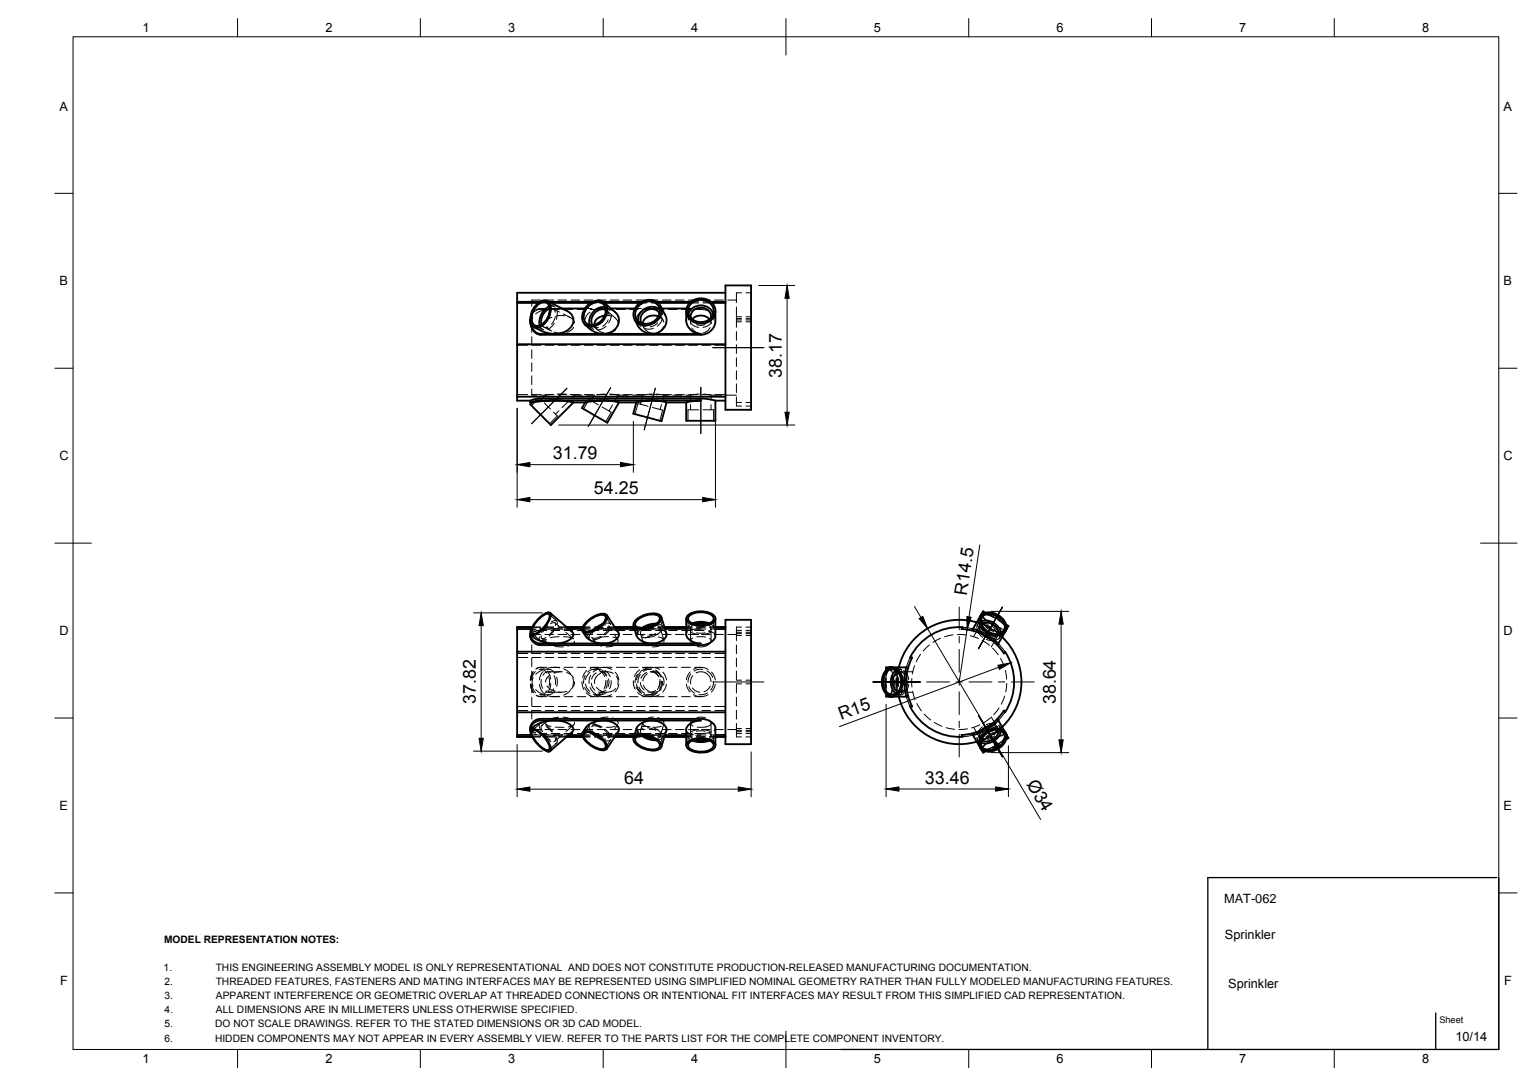
ISO-10303-21;
HEADER;
/* Generated by software containing ST-Developer
 * from STEP Tools, Inc. (www.steptools.com) 
 */

FILE_DESCRIPTION(
/* description */ (''),
/* implementation_level */ '2;1');

FILE_NAME(
/* name */ 'Sprinkler.step',
/* time_stamp */ '2026-10-24T10:18:25-07:00',
/* author */ (''),
/* organization */ (''),
/* preprocessor_version */ 'ST-DEVELOPER v20.2',
/* originating_system */ 'Autodesk Translation Framework v15.15.0.0',
/* authorisation */ '');

FILE_SCHEMA (('AUTOMOTIVE_DESIGN { 1 0 10303 214 3 1 1 }'));
ENDSEC;

DATA;
#10=MECHANICAL_DESIGN_GEOMETRIC_PRESENTATION_REPRESENTATION('',(#264),#14125);
#235=SHAPE_REPRESENTATION_RELATIONSHIP('SRR','None',#14209,#245);
#245=ADVANCED_BREP_SHAPE_REPRESENTATION('',(#277),#14123);
#264=STYLED_ITEM('',(#14263),#277);
#277=MANIFOLD_SOLID_BREP('Sprinkler',#6145);
#289=B_SPLINE_SURFACE_WITH_KNOTS('',3,1,((#13841,#13842),(#13843,#13844),
(#13845,#13846),(#13847,#13848),(#13849,#13850),(#13851,#13852),(#13853,
#13854),(#13855,#13856),(#13857,#13858),(#13859,#13860),(#13861,#13862)),
 .UNSPECIFIED.,.F.,.F.,.F.,(4,1,1,1,1,1,1,1,4),(2,2),(3.14159265358979,
3.53429173528852,3.92699081698724,4.31968989868597,4.71238898038469,5.10508806208341,
5.49778714378214,5.89048622548086,6.28318530717959),(0.,0.129347179873149),
 .UNSPECIFIED.);
#290=B_SPLINE_SURFACE_WITH_KNOTS('',3,1,((#13904,#13905),(#13906,#13907),
(#13908,#13909),(#13910,#13911),(#13912,#13913),(#13914,#13915),(#13916,
#13917),(#13918,#13919),(#13920,#13921),(#13922,#13923),(#13924,#13925)),
 .UNSPECIFIED.,.F.,.F.,.F.,(4,1,1,1,1,1,1,1,4),(2,2),(3.14159265358979,
3.53429173528851,3.92699081698724,4.31968989868596,4.71238898038469,5.10508806208341,
5.49778714378214,5.89048622548086,6.28318530717959),(0.,0.129347179873148),
 .UNSPECIFIED.);
#291=B_SPLINE_SURFACE_WITH_KNOTS('',3,1,((#13967,#13968),(#13969,#13970),
(#13971,#13972),(#13973,#13974),(#13975,#13976),(#13977,#13978),(#13979,
#13980),(#13981,#13982),(#13983,#13984),(#13985,#13986),(#13987,#13988)),
 .UNSPECIFIED.,.F.,.F.,.F.,(4,1,1,1,1,1,1,1,4),(2,2),(3.14159265358979,
3.53429173528851,3.92699081698723,4.31968989868596,4.71238898038468,5.10508806208341,
5.49778714378213,5.89048622548085,6.28318530717958),(0.,0.129347179873145),
 .UNSPECIFIED.);
#411=B_SPLINE_CURVE_WITH_KNOTS('',3,(#12350,#12351,#12352,#12353,#12354,
#12355,#12356,#12357),.UNSPECIFIED.,.F.,.F.,(4,2,2,4),(0.801601659973552,
0.908686694681274,1.06147652934293,1.21426636400458),.UNSPECIFIED.);
#412=B_SPLINE_CURVE_WITH_KNOTS('',3,(#12359,#12360,#12361,#12362,#12363,
#12364,#12365,#12366,#12367,#12368,#12369,#12370,#12371,#12372),
 .UNSPECIFIED.,.F.,.F.,(4,2,2,2,2,2,4),(0.,0.152789834661652,0.305579669323305,
0.456356425662796,0.607133182002287,0.757909938341781,0.801601659973552),
 .UNSPECIFIED.);
#413=B_SPLINE_CURVE_WITH_KNOTS('',3,(#12376,#12377,#12378,#12379,#12380,
#12381,#12382,#12383,#12384,#12385,#12386,#12387,#12388,#12389,#12390,#12391),
 .UNSPECIFIED.,.F.,.F.,(4,2,2,2,2,2,2,4),(1.41258149283994,1.51470567835646,
1.66615965590029,1.81761363344413,1.96906761098797,2.12052158853181,2.27200321656199,
2.42348484459217),.UNSPECIFIED.);
#414=B_SPLINE_CURVE_WITH_KNOTS('',3,(#12392,#12393,#12394,#12395,#12396,
#12397),.UNSPECIFIED.,.F.,.F.,(4,2,4),(1.21174242229609,1.36322405032627,
1.41258149283994),.UNSPECIFIED.);
#415=B_SPLINE_CURVE_WITH_KNOTS('',3,(#12402,#12403,#12404,#12405,#12406,
#12407,#12408,#12409),.UNSPECIFIED.,.F.,.F.,(4,2,2,4),(0.810459053731311,
0.931112082660273,1.09792489409666,1.26473770553305),.UNSPECIFIED.);
#416=B_SPLINE_CURVE_WITH_KNOTS('',3,(#12411,#12412,#12413,#12414,#12415,
#12416,#12417,#12418,#12419,#12420,#12421,#12422,#12423,#12424),
 .UNSPECIFIED.,.F.,.F.,(4,2,2,2,2,2,4),(0.,0.166812811436392,0.333625622872784,
0.482997237819655,0.632368852766526,0.781740467713401,0.810459053731311),
 .UNSPECIFIED.);
#417=B_SPLINE_CURVE_WITH_KNOTS('',3,(#12426,#12427,#12428,#12429,#12430,
#12431,#12432,#12433,#12434,#12435,#12436,#12437,#12438,#12439,#12440,#12441,
#12442,#12443),.UNSPECIFIED.,.F.,.F.,(4,2,2,2,2,2,2,2,4),(1.21426636400458,
1.37281902636882,1.53137168873306,1.68587949128402,1.84038729383497,1.99489509638593,
2.14940289893689,2.30795556130114,2.46650822366539),.UNSPECIFIED.);
#418=B_SPLINE_CURVE_WITH_KNOTS('',3,(#12448,#12449,#12450,#12451,#12452,
#12453,#12454,#12455,#12456,#12457),.UNSPECIFIED.,.F.,.F.,(4,2,2,2,4),(0.84921255840186,
0.855460999411689,1.0133776521287,1.20423317275903,1.39508869338936),
 .UNSPECIFIED.);
#419=B_SPLINE_CURVE_WITH_KNOTS('',3,(#12459,#12460,#12461,#12462,#12463,
#12464,#12465,#12466,#12467,#12468,#12469,#12470),.UNSPECIFIED.,.F.,.F.,
(4,2,2,2,2,4),(0.,0.19085552063033,0.38171104126066,0.539627693977667,0.697544346694674,
0.84921255840186),.UNSPECIFIED.);
#420=B_SPLINE_CURVE_WITH_KNOTS('',3,(#12472,#12473,#12474,#12475,#12476,
#12477,#12478,#12479,#12480,#12481,#12482,#12483,#12484,#12485,#12486,#12487,
#12488,#12489),.UNSPECIFIED.,.F.,.F.,(4,2,2,2,2,2,2,2,4),(1.26473770553305,
1.44115993597425,1.61758216641546,1.77878219205947,1.93998221770349,2.10118224334752,
2.26238226899155,2.43880449943275,2.61522672987395),.UNSPECIFIED.);
#421=B_SPLINE_CURVE_WITH_KNOTS('',3,(#12493,#12494,#12495,#12496,#12497,
#12498,#12499,#12500,#12501,#12502,#12503,#12504,#12505,#12506,#12507,#12508,
#12509,#12510,#12511,#12512,#12513,#12514),.UNSPECIFIED.,.F.,.F.,(4,2,2,
2,2,2,2,2,2,2,4),(1.39508869338936,1.63068735474474,1.86628601610013,2.01895939966093,
2.09529609144134,2.17163278322174,2.24796947500215,2.32430616678255,2.47697955034337,
2.71257821169876,2.94817687305416),.UNSPECIFIED.);
#422=B_SPLINE_CURVE_WITH_KNOTS('',3,(#12517,#12518,#12519,#12520,#12521,
#12522,#12523,#12524,#12525,#12526,#12527,#12528,#12529,#12530,#12531,#12532,
#12533,#12534,#12535,#12536,#12537,#12538,#12539,#12540,#12541,#12542),
 .UNSPECIFIED.,.F.,.F.,(4,2,2,2,2,2,2,2,2,2,2,2,4),(0.,0.0444658256706816,
0.109825747467382,0.210987273969983,0.363115011869221,0.476603266918211,
0.543343022865724,0.610052308554092,0.7232875236507,0.87579543247345,0.97697424211648,
1.04237097445545,1.08685368328188),.UNSPECIFIED.);
#423=B_SPLINE_CURVE_WITH_KNOTS('',3,(#12557,#12558,#12559,#12560,#12561,
#12562,#12563,#12564),.UNSPECIFIED.,.F.,.F.,(4,2,2,4),(0.801601659973551,
0.908686694681269,1.06147652934292,1.21426636400457),.UNSPECIFIED.);
#424=B_SPLINE_CURVE_WITH_KNOTS('',3,(#12566,#12567,#12568,#12569,#12570,
#12571,#12572,#12573,#12574,#12575,#12576,#12577,#12578,#12579),
 .UNSPECIFIED.,.F.,.F.,(4,2,2,2,2,2,4),(0.,0.152789834661651,0.305579669323302,
0.456356425662796,0.607133182002289,0.757909938341779,0.801601659973551),
 .UNSPECIFIED.);
#425=B_SPLINE_CURVE_WITH_KNOTS('',3,(#12583,#12584,#12585,#12586,#12587,
#12588,#12589,#12590,#12591,#12592,#12593,#12594,#12595,#12596,#12597,#12598),
 .UNSPECIFIED.,.F.,.F.,(4,2,2,2,2,2,2,4),(1.41258149283993,1.51470567835645,
1.66615965590029,1.81761363344413,1.96906761098797,2.1205215885318,2.27200321656199,
2.42348484459217),.UNSPECIFIED.);
#426=B_SPLINE_CURVE_WITH_KNOTS('',3,(#12599,#12600,#12601,#12602,#12603,
#12604),.UNSPECIFIED.,.F.,.F.,(4,2,4),(1.21174242229609,1.36322405032627,
1.41258149283993),.UNSPECIFIED.);
#427=B_SPLINE_CURVE_WITH_KNOTS('',3,(#12609,#12610,#12611,#12612,#12613,
#12614,#12615,#12616),.UNSPECIFIED.,.F.,.F.,(4,2,2,4),(0.810459053731318,
0.931112082660271,1.09792489409666,1.26473770553306),.UNSPECIFIED.);
#428=B_SPLINE_CURVE_WITH_KNOTS('',3,(#12618,#12619,#12620,#12621,#12622,
#12623,#12624,#12625,#12626,#12627,#12628,#12629,#12630,#12631),
 .UNSPECIFIED.,.F.,.F.,(4,2,2,2,2,2,4),(0.,0.166812811436393,0.333625622872785,
0.482997237819654,0.632368852766523,0.781740467713397,0.810459053731318),
 .UNSPECIFIED.);
#429=B_SPLINE_CURVE_WITH_KNOTS('',3,(#12633,#12634,#12635,#12636,#12637,
#12638,#12639,#12640,#12641,#12642,#12643,#12644,#12645,#12646,#12647,#12648,
#12649,#12650),.UNSPECIFIED.,.F.,.F.,(4,2,2,2,2,2,2,2,4),(1.21426636400457,
1.37281902636881,1.53137168873306,1.68587949128401,1.84038729383497,1.99489509638593,
2.14940289893689,2.30795556130114,2.46650822366538),.UNSPECIFIED.);
#430=B_SPLINE_CURVE_WITH_KNOTS('',3,(#12655,#12656,#12657,#12658,#12659,
#12660,#12661,#12662),.UNSPECIFIED.,.F.,.F.,(4,2,2,4),(0.848478832255458,
0.991796836691898,1.19347267089766,1.39514850510343),.UNSPECIFIED.);
#431=B_SPLINE_CURVE_WITH_KNOTS('',3,(#12664,#12665,#12666,#12667,#12668,
#12669,#12670,#12671,#12672,#12673,#12674,#12675,#12676,#12677),
 .UNSPECIFIED.,.F.,.F.,(4,2,2,2,2,2,4),(0.,0.201675834205757,0.403351668411514,
0.550462960481608,0.697574252551703,0.8446855446218,0.848478832255458),
 .UNSPECIFIED.);
#432=B_SPLINE_CURVE_WITH_KNOTS('',3,(#12679,#12680,#12681,#12682,#12683,
#12684,#12685,#12686,#12687,#12688,#12689,#12690,#12691,#12692,#12693,#12694,
#12695,#12696),.UNSPECIFIED.,.F.,.F.,(4,2,2,2,2,2,2,2,4),(1.26473770553306,
1.44115993597426,1.61758216641546,1.77878219205948,1.93998221770349,2.10118224334752,
2.26238226899154,2.43880449943275,2.61522672987395),.UNSPECIFIED.);
#433=B_SPLINE_CURVE_WITH_KNOTS('',3,(#12700,#12701,#12702,#12703,#12704,
#12705,#12706,#12707,#12708,#12709,#12710,#12711,#12712,#12713,#12714,#12715,
#12716,#12717,#12718,#12719,#12720,#12721),.UNSPECIFIED.,.F.,.F.,(4,2,2,
2,2,2,2,2,2,2,4),(1.39514850510343,1.60860320712188,1.82205790914033,1.99791237111712,
2.08583960210551,2.17376683309391,2.26169406408231,2.34962129507071,2.5254757570475,
2.73893045906596,2.95238516108442),.UNSPECIFIED.);
#434=B_SPLINE_CURVE_WITH_KNOTS('',3,(#12724,#12725,#12726,#12727,#12728,
#12729,#12730,#12731,#12732,#12733,#12734,#12735,#12736,#12737,#12738,#12739,
#12740,#12741,#12742,#12743,#12744,#12745,#12746,#12747,#12748,#12749),
 .UNSPECIFIED.,.F.,.F.,(4,2,2,2,2,2,2,2,2,2,2,2,4),(0.,0.0444658256707017,
0.109825747467453,0.210987273970143,0.363115011869592,0.4766032669186,0.543343022866364,
0.610052308555067,0.723287523653244,0.875795432478097,0.97697424212264,
1.04237097446268,1.08685368328966),.UNSPECIFIED.);
#435=B_SPLINE_CURVE_WITH_KNOTS('',3,(#12755,#12756,#12757,#12758,#12759,
#12760,#12761,#12762),.UNSPECIFIED.,.F.,.F.,(4,2,2,4),(0.80160165997355,
0.908686694681275,1.06147652934293,1.21426636400458),.UNSPECIFIED.);
#436=B_SPLINE_CURVE_WITH_KNOTS('',3,(#12764,#12765,#12766,#12767,#12768,
#12769,#12770,#12771,#12772,#12773,#12774,#12775,#12776,#12777),
 .UNSPECIFIED.,.F.,.F.,(4,2,2,2,2,2,4),(0.,0.152789834661653,0.305579669323305,
0.456356425662799,0.607133182002292,0.757909938341784,0.80160165997355),
 .UNSPECIFIED.);
#437=B_SPLINE_CURVE_WITH_KNOTS('',3,(#12781,#12782,#12783,#12784,#12785,
#12786,#12787,#12788,#12789,#12790,#12791,#12792,#12793,#12794,#12795,#12796),
 .UNSPECIFIED.,.F.,.F.,(4,2,2,2,2,2,2,4),(1.41258149283993,1.51470567835645,
1.66615965590029,1.81761363344413,1.96906761098797,2.12052158853181,2.27200321656199,
2.42348484459217),.UNSPECIFIED.);
#438=B_SPLINE_CURVE_WITH_KNOTS('',3,(#12797,#12798,#12799,#12800,#12801,
#12802),.UNSPECIFIED.,.F.,.F.,(4,2,4),(1.21174242229609,1.36322405032627,
1.41258149283993),.UNSPECIFIED.);
#439=B_SPLINE_CURVE_WITH_KNOTS('',3,(#12807,#12808,#12809,#12810,#12811,
#12812,#12813,#12814),.UNSPECIFIED.,.F.,.F.,(4,2,2,4),(0.810451797988797,
0.931104826917751,1.09791763835414,1.26473044979053),.UNSPECIFIED.);
#440=B_SPLINE_CURVE_WITH_KNOTS('',3,(#12816,#12817,#12818,#12819,#12820,
#12821,#12822,#12823,#12824,#12825,#12826,#12827,#12828,#12829),
 .UNSPECIFIED.,.F.,.F.,(4,2,2,2,2,2,4),(0.,0.163827053405726,0.327654106811452,
0.48000785191773,0.632361597024009,0.781733211970881,0.810451797988797),
 .UNSPECIFIED.);
#441=B_SPLINE_CURVE_WITH_KNOTS('',3,(#12831,#12832,#12833,#12834,#12835,
#12836,#12837,#12838,#12839,#12840,#12841,#12842,#12843,#12844,#12845,#12846,
#12847,#12848),.UNSPECIFIED.,.F.,.F.,(4,2,2,2,2,2,2,2,4),(1.21426636400458,
1.37281902636882,1.53137168873306,1.68587949128402,1.84038729383497,1.99489509638594,
2.1494028989369,2.30795556130114,2.46650822366539),.UNSPECIFIED.);
#442=B_SPLINE_CURVE_WITH_KNOTS('',3,(#12853,#12854,#12855,#12856,#12857,
#12858,#12859,#12860,#12861,#12862),.UNSPECIFIED.,.F.,.F.,(4,2,2,2,4),(0.849212558401863,
0.855460999411694,1.01337765212871,1.20423317275904,1.39508869338936),
 .UNSPECIFIED.);
#443=B_SPLINE_CURVE_WITH_KNOTS('',3,(#12864,#12865,#12866,#12867,#12868,
#12869,#12870,#12871,#12872,#12873,#12874,#12875),.UNSPECIFIED.,.F.,.F.,
(4,2,2,2,2,4),(0.,0.190855520630331,0.381711041260663,0.539627693977671,
0.697544346694678,0.849212558401863),.UNSPECIFIED.);
#444=B_SPLINE_CURVE_WITH_KNOTS('',3,(#12877,#12878,#12879,#12880,#12881,
#12882,#12883,#12884,#12885,#12886,#12887,#12888,#12889,#12890,#12891,#12892,
#12893,#12894),.UNSPECIFIED.,.F.,.F.,(4,2,2,2,2,2,2,2,4),(1.26473044979053,
1.45047293867533,1.63621542756013,1.78793284105988,1.93965025455964,2.0913676680594,
2.24308508155916,2.42882757044396,2.61457005932877),.UNSPECIFIED.);
#445=B_SPLINE_CURVE_WITH_KNOTS('',3,(#12898,#12899,#12900,#12901,#12902,
#12903,#12904,#12905,#12906,#12907,#12908,#12909,#12910,#12911,#12912,#12913,
#12914,#12915,#12916,#12917,#12918,#12919),.UNSPECIFIED.,.F.,.F.,(4,2,2,
2,2,2,2,2,2,2,4),(1.39508869338936,1.63068735474475,1.86628601610013,2.01895939966094,
2.09529609144135,2.17163278322175,2.24796947500216,2.32430616678257,2.47697955034339,
2.71257821169878,2.94817687305417),.UNSPECIFIED.);
#446=B_SPLINE_CURVE_WITH_KNOTS('',3,(#12922,#12923,#12924,#12925,#12926,
#12927,#12928,#12929,#12930,#12931,#12932,#12933,#12934,#12935,#12936,#12937,
#12938,#12939,#12940,#12941,#12942,#12943,#12944,#12945,#12946,#12947),
 .UNSPECIFIED.,.F.,.F.,(4,2,2,2,2,2,2,2,2,2,2,2,4),(0.,0.0444658256707104,
0.109825747467599,0.210987273970278,0.3631150118696,0.476603266918339,0.54334302286555,
0.610052308553677,0.723287523650531,0.875795432473984,0.97697424211741,
1.0423709744566,1.08685368328313),.UNSPECIFIED.);
#447=B_SPLINE_CURVE_WITH_KNOTS('',3,(#13048,#13049,#13050,#13051,#13052,
#13053,#13054,#13055,#13056,#13057,#13058,#13059,#13060,#13061,#13062,#13063,
#13064,#13065),.UNSPECIFIED.,.F.,.F.,(4,2,2,2,2,2,2,2,4),(-2.42440986895006,
-2.27286833474306,-2.12132680053607,-1.9698171011243,-1.81830740171254,
-1.66679770230078,-1.51528800288901,-1.36374646868202,-1.21220493447502),
 .UNSPECIFIED.);
#448=B_SPLINE_CURVE_WITH_KNOTS('',3,(#13115,#13116,#13117,#13118,#13119,
#13120,#13121,#13122,#13123,#13124,#13125,#13126,#13127,#13128,#13129,#13130,
#13131,#13132,#13133,#13134,#13135),.UNSPECIFIED.,.F.,.F.,(4,2,2,2,3,2,
2,2,2,4),(1.63431795680218,1.63484051213071,1.74655213492763,1.90358589296679,
2.06061965100595,2.19559646985844,2.33057328871092,2.44200600177385,2.55343871483678,
2.66004451397958),.UNSPECIFIED.);
#449=B_SPLINE_CURVE_WITH_KNOTS('',3,(#13136,#13137,#13138,#13139,#13140,
#13141,#13142,#13143,#13144,#13145,#13146,#13147,#13148,#13149,#13150,#13151,
#13152,#13153,#13154,#13155,#13156,#13157,#13158,#13159),.UNSPECIFIED.,
 .F.,.F.,(4,2,2,2,2,2,2,2,2,2,2,4),(2.66004451397958,2.66487142789972,2.77630414096266,
2.91128095981515,3.04625777866764,3.20329153670679,3.36032529474595,3.47203691754285,
3.5278927289413,3.58374854033975,3.63960435173821,3.69493760780813),
 .UNSPECIFIED.);
#450=B_SPLINE_CURVE_WITH_KNOTS('',3,(#13162,#13163,#13164,#13165,#13166,
#13167,#13168,#13169,#13170,#13171,#13172,#13173,#13174,#13175,#13176,#13177,
#13178,#13179,#13180,#13181,#13182,#13183,#13184),.UNSPECIFIED.,.F.,.F.,
(4,2,2,2,3,2,2,2,2,2,4),(1.63645246149242,1.6458071028209,1.76735674157733,
1.91500283165642,2.06264892173552,2.21065304350676,2.35865716527801,2.45711954510512,
2.55558192493224,2.65404430475936,2.66124396153498),.UNSPECIFIED.);
#451=B_SPLINE_CURVE_WITH_KNOTS('',3,(#13185,#13186,#13187,#13188,#13189,
#13190,#13191,#13192,#13193,#13194,#13195,#13196,#13197,#13198,#13199,#13200,
#13201,#13202,#13203,#13204,#13205,#13206),.UNSPECIFIED.,.F.,.F.,(4,2,2,
2,2,2,2,2,2,2,4),(2.66124396153498,2.75250668458648,2.90051080635773,3.04851492812899,
3.19616101820807,3.34380710828715,3.46535674704357,3.52613156642178,3.58690638579999,
3.64768120517821,3.69910138322794),.UNSPECIFIED.);
#452=B_SPLINE_CURVE_WITH_KNOTS('',3,(#13209,#13210,#13211,#13212,#13213,
#13214,#13215,#13216,#13217,#13218,#13219,#13220,#13221,#13222,#13223,#13224,
#13225,#13226,#13227,#13228,#13229),.UNSPECIFIED.,.F.,.F.,(4,2,2,3,2,2,
2,2,2,4),(1.48658026968319,1.57668032617585,1.70181043495793,1.82694054374001,
1.94229840394621,2.0576562641524,2.16466765320846,2.27167904226452,2.37869043132058,
2.39673280800115),.UNSPECIFIED.);
#453=B_SPLINE_CURVE_WITH_KNOTS('',3,(#13230,#13231,#13232,#13233,#13234,
#13235,#13236,#13237,#13238,#13239,#13240,#13241,#13242,#13243,#13244,#13245,
#13246,#13247,#13248,#13249),.UNSPECIFIED.,.F.,.F.,(4,2,2,2,2,2,2,2,2,4),
(2.39673280800115,2.48570182037664,2.60105968058284,2.71641754078903,2.84154764957111,
2.96667775835319,3.07591353624385,3.18514931413451,3.29438509202518,3.3135208134232),
 .UNSPECIFIED.);
#454=B_SPLINE_CURVE_WITH_KNOTS('',3,(#13252,#13253,#13254,#13255,#13256,
#13257,#13258,#13259,#13260,#13261,#13262,#13263,#13264,#13265,#13266,#13267,
#13268,#13269,#13270,#13271,#13272),.UNSPECIFIED.,.F.,.F.,(4,2,2,3,2,2,
2,2,2,4),(1.48667142164751,1.57677147814025,1.70190158692234,1.82703169570442,
1.94802136665288,2.06901103760135,2.17041340390623,2.27181577021112,2.37321813651602,
2.39644556681379),.UNSPECIFIED.);
#455=B_SPLINE_CURVE_WITH_KNOTS('',3,(#13273,#13274,#13275,#13276,#13277,
#13278,#13279,#13280,#13281,#13282,#13283,#13284,#13285,#13286,#13287,#13288,
#13289,#13290,#13291,#13292),.UNSPECIFIED.,.F.,.F.,(4,2,2,2,2,2,2,2,2,4),
(2.39644556681379,2.47462050282091,2.59561017376938,2.71659984471785,2.84172995349992,
2.966860062282,3.07609584017266,3.18533161806333,3.294567395954,3.31370311735193),
 .UNSPECIFIED.);
#456=B_SPLINE_CURVE_WITH_KNOTS('',3,(#13295,#13296,#13297,#13298,#13299,
#13300,#13301,#13302,#13303,#13304,#13305,#13306,#13307,#13308,#13309,#13310,
#13311,#13312,#13313,#13314,#13315),.UNSPECIFIED.,.F.,.F.,(4,2,2,3,2,2,
2,2,2,4),(1.42510602309759,1.50257240162674,1.61295870334865,1.72334500507057,
1.83225417045197,1.94116333583337,2.04500754168813,2.1488517475429,2.25269595339766,
2.2848744256183),.UNSPECIFIED.);
#457=B_SPLINE_CURVE_WITH_KNOTS('',3,(#13316,#13317,#13318,#13319,#13320,
#13321,#13322,#13323,#13324,#13325,#13326,#13327,#13328,#13329,#13330,#13331,
#13332,#13333,#13334,#13335),.UNSPECIFIED.,.F.,.F.,(4,2,2,2,2,2,2,2,2,4),
(2.2848744256183,2.35654015925242,2.46544932463382,2.57435849001523,2.68474479173714,
2.79513109345905,2.90282767176861,3.01052425007817,3.11822082838774,3.14845102816816),
 .UNSPECIFIED.);
#458=B_SPLINE_CURVE_WITH_KNOTS('',3,(#13338,#13339,#13340,#13341,#13342,
#13343,#13344,#13345,#13346,#13347,#13348,#13349,#13350,#13351,#13352,#13353,
#13354,#13355,#13356,#13357,#13358),.UNSPECIFIED.,.F.,.F.,(4,2,2,3,2,2,
2,2,2,4),(1.42506934481542,1.50220099251643,1.61276096598296,1.72332093944948,
1.83050112648501,1.93768131352053,2.04324956210919,2.14881781069785,2.25438605928651,
2.28497277338716),.UNSPECIFIED.);
#459=B_SPLINE_CURVE_WITH_KNOTS('',3,(#13359,#13360,#13361,#13362,#13363,
#13364,#13365,#13366,#13367,#13368,#13369,#13370,#13371,#13372,#13373,#13374,
#13375,#13376,#13377,#13378),.UNSPECIFIED.,.F.,.F.,(4,2,2,2,2,2,2,2,2,4),
(2.28497277338716,2.35995430787517,2.46713449491069,2.57431468194622,2.68487465541274,
2.79543462887926,2.90295645465092,3.01047828042258,3.11800010619425,3.1483902842649),
 .UNSPECIFIED.);
#460=B_SPLINE_CURVE_WITH_KNOTS('',3,(#13381,#13382,#13383,#13384,#13385,
#13386,#13387,#13388,#13389,#13390,#13391,#13392,#13393,#13394,#13395,#13396,
#13397,#13398,#13399,#13400),.UNSPECIFIED.,.F.,.F.,(4,2,2,2,2,2,2,2,2,4),
(0.140389663816896,0.211667950083815,0.317493899242379,0.423319848400943,
0.529145797559505,0.634971746718067,0.740805721759974,0.846639696801881,
0.952473671843789,0.987029360618753),.UNSPECIFIED.);
#461=B_SPLINE_CURVE_WITH_KNOTS('',3,(#13401,#13402,#13403,#13404,#13405,
#13406,#13407,#13408,#13409,#13410,#13411,#13412,#13413,#13414,#13415,#13416,
#13417,#13418,#13419,#13420,#13421),.UNSPECIFIED.,.F.,.F.,(4,2,2,2,2,2,
2,3,2,4),(0.987029360618753,1.0583076468857,1.16413359604426,1.26995954520282,
1.37578549436138,1.48161144351995,1.58744541856186,1.69327939360377,1.79911336864567,
1.83366905742066),.UNSPECIFIED.);
#462=B_SPLINE_CURVE_WITH_KNOTS('',3,(#13424,#13425,#13426,#13427,#13428,
#13429,#13430,#13431,#13432,#13433,#13434,#13435,#13436,#13437,#13438,#13439,
#13440,#13441,#13442,#13443),.UNSPECIFIED.,.F.,.F.,(4,2,2,2,2,2,2,2,2,4),
(0.14038966381692,0.211667950083817,0.317493899242381,0.423319848400946,
0.529145797559508,0.634971746718069,0.740805721759977,0.846639696801884,
0.952473671843792,0.987029360618756),.UNSPECIFIED.);
#463=B_SPLINE_CURVE_WITH_KNOTS('',3,(#13444,#13445,#13446,#13447,#13448,
#13449,#13450,#13451,#13452,#13453,#13454,#13455,#13456,#13457,#13458,#13459,
#13460,#13461,#13462,#13463,#13464),.UNSPECIFIED.,.F.,.F.,(4,2,2,2,2,2,
2,3,2,4),(0.987029360618756,1.0583076468857,1.16413359604426,1.26995954520282,
1.37578549436139,1.48161144351995,1.58744541856186,1.69327939360377,1.79911336864568,
1.83366905742069),.UNSPECIFIED.);
#464=B_SPLINE_CURVE_WITH_KNOTS('',3,(#13467,#13468,#13469,#13470,#13471,
#13472,#13473,#13474,#13475,#13476,#13477,#13478,#13479,#13480,#13481,#13482,
#13483,#13484,#13485,#13486,#13487),.UNSPECIFIED.,.F.,.F.,(4,2,2,2,3,2,
2,2,2,4),(1.63431795680214,1.63484051213073,1.74655213492764,1.90358589296679,
2.06061965100595,2.19559646985844,2.33057328871092,2.44200600177386,2.5534387148368,
2.66004451397959),.UNSPECIFIED.);
#465=B_SPLINE_CURVE_WITH_KNOTS('',3,(#13488,#13489,#13490,#13491,#13492,
#13493,#13494,#13495,#13496,#13497,#13498,#13499,#13500,#13501,#13502,#13503,
#13504,#13505,#13506,#13507,#13508,#13509,#13510,#13511),.UNSPECIFIED.,
 .F.,.F.,(4,2,2,2,2,2,2,2,2,2,2,4),(2.66004451397959,2.66487142789973,2.77630414096267,
2.91128095981515,3.04625777866764,3.2032915367068,3.36032529474595,3.47203691754286,
3.52789272894132,3.58374854033977,3.63960435173823,3.69493760780809),
 .UNSPECIFIED.);
#466=B_SPLINE_CURVE_WITH_KNOTS('',3,(#13514,#13515,#13516,#13517,#13518,
#13519,#13520,#13521,#13522,#13523,#13524,#13525,#13526,#13527,#13528,#13529,
#13530,#13531,#13532,#13533,#13534),.UNSPECIFIED.,.F.,.F.,(4,2,2,3,2,2,
2,2,2,4),(1.48658026968317,1.57668032617585,1.70181043495793,1.82694054374001,
1.9422984039462,2.0576562641524,2.16466765320846,2.27167904226452,2.37869043132058,
2.39673280800115),.UNSPECIFIED.);
#467=B_SPLINE_CURVE_WITH_KNOTS('',3,(#13535,#13536,#13537,#13538,#13539,
#13540,#13541,#13542,#13543,#13544,#13545,#13546,#13547,#13548,#13549,#13550,
#13551,#13552,#13553,#13554),.UNSPECIFIED.,.F.,.F.,(4,2,2,2,2,2,2,2,2,4),
(2.39673280800115,2.48570182037664,2.60105968058283,2.71641754078903,2.84154764957111,
2.96667775835319,3.07591353624386,3.18514931413453,3.29438509202519,3.31352081342317),
 .UNSPECIFIED.);
#468=B_SPLINE_CURVE_WITH_KNOTS('',3,(#13557,#13558,#13559,#13560,#13561,
#13562,#13563,#13564,#13565,#13566,#13567,#13568,#13569,#13570,#13571,#13572,
#13573,#13574,#13575,#13576,#13577),.UNSPECIFIED.,.F.,.F.,(4,2,2,3,2,2,
2,2,2,4),(1.42506934481545,1.50220099251643,1.61276096598296,1.72332093944948,
1.83050112648501,1.93768131352053,2.04324956210919,2.14881781069785,2.25438605928651,
2.28497277338716),.UNSPECIFIED.);
#469=B_SPLINE_CURVE_WITH_KNOTS('',3,(#13578,#13579,#13580,#13581,#13582,
#13583,#13584,#13585,#13586,#13587,#13588,#13589,#13590,#13591,#13592,#13593,
#13594,#13595,#13596,#13597),.UNSPECIFIED.,.F.,.F.,(4,2,2,2,2,2,2,2,2,4),
(2.28497277338716,2.35995430787516,2.46713449491069,2.57431468194622,2.68487465541274,
2.79543462887926,2.90295645465092,3.01047828042259,3.11800010619425,3.14839028426493),
 .UNSPECIFIED.);
#470=B_SPLINE_CURVE_WITH_KNOTS('',3,(#13600,#13601,#13602,#13603,#13604,
#13605,#13606,#13607,#13608,#13609,#13610,#13611,#13612,#13613,#13614,#13615,
#13616,#13617,#13618,#13619),.UNSPECIFIED.,.F.,.F.,(4,2,2,2,2,2,2,2,2,4),
(0.140389663816901,0.211667950083817,0.31749389924238,0.423319848400942,
0.529145797559504,0.634971746718067,0.740805721759975,0.846639696801883,
0.952473671843791,0.987029360618755),.UNSPECIFIED.);
#471=B_SPLINE_CURVE_WITH_KNOTS('',3,(#13620,#13621,#13622,#13623,#13624,
#13625,#13626,#13627,#13628,#13629,#13630,#13631,#13632,#13633,#13634,#13635,
#13636,#13637,#13638,#13639,#13640),.UNSPECIFIED.,.F.,.F.,(4,2,2,2,2,2,
2,3,2,4),(0.987029360618755,1.0583076468857,1.16413359604426,1.26995954520283,
1.37578549436139,1.48161144351995,1.58744541856186,1.69327939360377,1.79911336864568,
1.83366905742067),.UNSPECIFIED.);
#472=B_SPLINE_CURVE_WITH_KNOTS('',3,(#13667,#13668,#13669,#13670,#13671,
#13672,#13673,#13674,#13675,#13676,#13677,#13678,#13679,#13680,#13681,#13682,
#13683,#13684),.UNSPECIFIED.,.F.,.F.,(4,2,2,2,2,2,2,2,4),(-2.42440986895005,
-2.27286833474305,-2.12132680053606,-1.96981710112429,-1.81830740171253,
-1.66679770230077,-1.51528800288901,-1.36374646868202,-1.21220493447502),
 .UNSPECIFIED.);
#473=B_SPLINE_CURVE_WITH_KNOTS('',3,(#13696,#13697,#13698,#13699,#13700,
#13701,#13702,#13703,#13704,#13705,#13706,#13707,#13708,#13709,#13710,#13711,
#13712,#13713),.UNSPECIFIED.,.F.,.F.,(4,2,2,2,2,2,2,2,4),(-2.42440986895003,
-2.27286833474304,-2.12132680053605,-1.96981710112428,-1.81830740171252,
-1.66679770230076,-1.515288002889,-1.36374646868201,-1.21220493447502),
 .UNSPECIFIED.);
#474=B_SPLINE_CURVE_WITH_KNOTS('',3,(#13863,#13864,#13865,#13866,#13867,
#13868,#13869,#13870,#13871,#13872,#13873,#13874,#13875,#13876,#13877,#13878,
#13879,#13880,#13881,#13882,#13883,#13884,#13885,#13886,#13887,#13888,#13889,
#13890),.UNSPECIFIED.,.F.,.F.,(4,2,2,2,2,2,2,2,2,2,2,2,2,4),(-1.08391055751389,
-1.04041495858034,-0.976127049627852,-0.875975346180159,-0.713802892781725,
-0.606446034139209,-0.5422685089836,-0.478121096415875,-0.370996668444261,
-0.213675448646841,-0.11261366027741,-0.0448303332672381,-0.0212473968071398,
0.),.UNSPECIFIED.);
#475=B_SPLINE_CURVE_WITH_KNOTS('',3,(#13926,#13927,#13928,#13929,#13930,
#13931,#13932,#13933,#13934,#13935,#13936,#13937,#13938,#13939,#13940,#13941,
#13942,#13943,#13944,#13945,#13946,#13947,#13948,#13949,#13950,#13951,#13952,
#13953),.UNSPECIFIED.,.F.,.F.,(4,2,2,2,2,2,2,2,2,2,2,2,2,4),(-1.08391055750046,
-1.04041495856732,-0.976127049615459,-0.875975346168904,-0.713802892772233,
-0.606446034130957,-0.542268508976211,-0.478121096409307,-0.370996668439296,
-0.213675448644088,-0.112613660276149,-0.0448303332669679,-0.0212473968071859,
0.),.UNSPECIFIED.);
#476=B_SPLINE_CURVE_WITH_KNOTS('',3,(#13989,#13990,#13991,#13992,#13993,
#13994,#13995,#13996,#13997,#13998,#13999,#14000,#14001,#14002,#14003,#14004,
#14005,#14006,#14007,#14008,#14009,#14010,#14011,#14012,#14013,#14014,#14015,
#14016),.UNSPECIFIED.,.F.,.F.,(4,2,2,2,2,2,2,2,2,2,2,2,2,4),(-1.0839105575165,
-1.04041495858262,-0.976127049629671,-0.8759753461813,-0.713802892781876,
-0.606446034138857,-0.542268508983049,-0.478121096415206,-0.370996668443923,
-0.21367544864674,-0.112613660277534,-0.0448303332674202,-0.021247396807171,
0.),.UNSPECIFIED.);
#566=CYLINDRICAL_SURFACE('',#6670,15.);
#567=CYLINDRICAL_SURFACE('',#6673,15.);
#568=CYLINDRICAL_SURFACE('',#6676,15.);
#569=CYLINDRICAL_SURFACE('',#6679,15.);
#570=CYLINDRICAL_SURFACE('',#6680,15.);
#571=CYLINDRICAL_SURFACE('',#6681,15.);
#572=CYLINDRICAL_SURFACE('',#6682,15.);
#573=CYLINDRICAL_SURFACE('',#6683,15.);
#574=CYLINDRICAL_SURFACE('',#6686,15.);
#575=CYLINDRICAL_SURFACE('',#6687,15.);
#576=CYLINDRICAL_SURFACE('',#6688,15.);
#577=CYLINDRICAL_SURFACE('',#6689,15.);
#578=CYLINDRICAL_SURFACE('',#6690,15.);
#579=CYLINDRICAL_SURFACE('',#6691,15.);
#580=CYLINDRICAL_SURFACE('',#6692,15.);
#581=CYLINDRICAL_SURFACE('',#6693,15.);
#582=CYLINDRICAL_SURFACE('',#6694,15.);
#583=CYLINDRICAL_SURFACE('',#6697,15.);
#584=CYLINDRICAL_SURFACE('',#6707,17.);
#585=CYLINDRICAL_SURFACE('',#6717,4.00000000000012);
#586=CYLINDRICAL_SURFACE('',#6721,4.00000000000001);
#587=CYLINDRICAL_SURFACE('',#6725,4.00000000000001);
#588=CYLINDRICAL_SURFACE('',#6729,4.);
#589=CYLINDRICAL_SURFACE('',#6733,3.50000000000012);
#590=CYLINDRICAL_SURFACE('',#6737,3.5);
#591=CYLINDRICAL_SURFACE('',#6741,3.49999999999992);
#592=CYLINDRICAL_SURFACE('',#6742,12.9999999999984);
#593=CYLINDRICAL_SURFACE('',#6748,3.49999999999998);
#594=CYLINDRICAL_SURFACE('',#6749,2.80000000000012);
#595=CYLINDRICAL_SURFACE('',#6750,2.79999999999998);
#596=CYLINDRICAL_SURFACE('',#6751,2.79999999999991);
#597=CYLINDRICAL_SURFACE('',#6752,2.79999999999999);
#598=CYLINDRICAL_SURFACE('',#6756,4.00000000000012);
#599=CYLINDRICAL_SURFACE('',#6760,4.00000000000012);
#600=CYLINDRICAL_SURFACE('',#6764,4.00000000000001);
#601=CYLINDRICAL_SURFACE('',#6768,4.00000000000001);
#602=CYLINDRICAL_SURFACE('',#6772,4.00000000000001);
#603=CYLINDRICAL_SURFACE('',#6776,4.00000000000001);
#604=CYLINDRICAL_SURFACE('',#6780,4.);
#605=CYLINDRICAL_SURFACE('',#6784,4.);
#606=CYLINDRICAL_SURFACE('',#6785,2.80000000000012);
#607=CYLINDRICAL_SURFACE('',#6787,2.80000000000012);
#608=CYLINDRICAL_SURFACE('',#6789,2.79999999999998);
#609=CYLINDRICAL_SURFACE('',#6791,2.79999999999998);
#610=CYLINDRICAL_SURFACE('',#6793,2.79999999999991);
#611=CYLINDRICAL_SURFACE('',#6795,2.79999999999991);
#612=CYLINDRICAL_SURFACE('',#6797,2.79999999999999);
#613=CYLINDRICAL_SURFACE('',#6799,2.79999999999999);
#614=CYLINDRICAL_SURFACE('',#6803,3.50000000000012);
#615=CYLINDRICAL_SURFACE('',#6806,3.50000000000012);
#616=CYLINDRICAL_SURFACE('',#6809,3.5);
#617=CYLINDRICAL_SURFACE('',#6812,3.5);
#618=CYLINDRICAL_SURFACE('',#6815,3.49999999999992);
#619=CYLINDRICAL_SURFACE('',#6818,3.49999999999992);
#620=CYLINDRICAL_SURFACE('',#6821,3.49999999999998);
#621=CYLINDRICAL_SURFACE('',#6824,3.49999999999998);
#622=CYLINDRICAL_SURFACE('',#6829,14.5);
#623=CYLINDRICAL_SURFACE('',#6834,14.5);
#624=CYLINDRICAL_SURFACE('',#6839,14.5);
#687=FACE_BOUND('',#1399,.T.);
#688=FACE_BOUND('',#1401,.T.);
#689=FACE_BOUND('',#1404,.T.);
#690=FACE_BOUND('',#1407,.T.);
#691=FACE_BOUND('',#1410,.T.);
#692=FACE_BOUND('',#1413,.T.);
#693=FACE_BOUND('',#1416,.T.);
#694=FACE_BOUND('',#1419,.T.);
#695=FACE_BOUND('',#1422,.T.);
#696=FACE_BOUND('',#1425,.T.);
#697=FACE_BOUND('',#1428,.T.);
#698=FACE_BOUND('',#1429,.T.);
#699=FACE_BOUND('',#1430,.T.);
#700=FACE_BOUND('',#1431,.T.);
#701=FACE_BOUND('',#1432,.T.);
#702=FACE_BOUND('',#1433,.T.);
#703=FACE_BOUND('',#1434,.T.);
#704=FACE_BOUND('',#1435,.T.);
#705=FACE_BOUND('',#1436,.T.);
#706=FACE_BOUND('',#1437,.T.);
#707=FACE_BOUND('',#1438,.T.);
#708=FACE_BOUND('',#1439,.T.);
#709=FACE_BOUND('',#1442,.T.);
#710=FACE_BOUND('',#1449,.T.);
#711=FACE_BOUND('',#1452,.T.);
#712=FACE_BOUND('',#1455,.T.);
#713=FACE_BOUND('',#1458,.T.);
#714=FACE_BOUND('',#1461,.T.);
#715=FACE_BOUND('',#1464,.T.);
#716=FACE_BOUND('',#1467,.T.);
#717=FACE_BOUND('',#1470,.T.);
#718=FACE_BOUND('',#1481,.T.);
#719=FACE_BOUND('',#1484,.T.);
#720=FACE_BOUND('',#1487,.T.);
#721=FACE_BOUND('',#1490,.T.);
#722=FACE_BOUND('',#1493,.T.);
#723=FACE_BOUND('',#1496,.T.);
#724=FACE_BOUND('',#1499,.T.);
#725=FACE_BOUND('',#1502,.T.);
#726=FACE_BOUND('',#1510,.T.);
#727=FACE_BOUND('',#1517,.T.);
#728=FACE_BOUND('',#1524,.T.);
#967=FACE_OUTER_BOUND('',#1380,.T.);
#968=FACE_OUTER_BOUND('',#1381,.T.);
#969=FACE_OUTER_BOUND('',#1382,.T.);
#970=FACE_OUTER_BOUND('',#1383,.T.);
#971=FACE_OUTER_BOUND('',#1384,.T.);
#972=FACE_OUTER_BOUND('',#1385,.T.);
#973=FACE_OUTER_BOUND('',#1386,.T.);
#974=FACE_OUTER_BOUND('',#1387,.T.);
#975=FACE_OUTER_BOUND('',#1388,.T.);
#976=FACE_OUTER_BOUND('',#1389,.T.);
#977=FACE_OUTER_BOUND('',#1390,.T.);
#978=FACE_OUTER_BOUND('',#1391,.T.);
#979=FACE_OUTER_BOUND('',#1392,.T.);
#980=FACE_OUTER_BOUND('',#1393,.T.);
#981=FACE_OUTER_BOUND('',#1394,.T.);
#982=FACE_OUTER_BOUND('',#1395,.T.);
#983=FACE_OUTER_BOUND('',#1396,.T.);
#984=FACE_OUTER_BOUND('',#1397,.T.);
#985=FACE_OUTER_BOUND('',#1398,.T.);
#986=FACE_OUTER_BOUND('',#1400,.T.);
#987=FACE_OUTER_BOUND('',#1402,.T.);
#988=FACE_OUTER_BOUND('',#1403,.T.);
#989=FACE_OUTER_BOUND('',#1405,.T.);
#990=FACE_OUTER_BOUND('',#1406,.T.);
#991=FACE_OUTER_BOUND('',#1408,.T.);
#992=FACE_OUTER_BOUND('',#1409,.T.);
#993=FACE_OUTER_BOUND('',#1411,.T.);
#994=FACE_OUTER_BOUND('',#1412,.T.);
#995=FACE_OUTER_BOUND('',#1414,.T.);
#996=FACE_OUTER_BOUND('',#1415,.T.);
#997=FACE_OUTER_BOUND('',#1417,.T.);
#998=FACE_OUTER_BOUND('',#1418,.T.);
#999=FACE_OUTER_BOUND('',#1420,.T.);
#1000=FACE_OUTER_BOUND('',#1421,.T.);
#1001=FACE_OUTER_BOUND('',#1423,.T.);
#1002=FACE_OUTER_BOUND('',#1424,.T.);
#1003=FACE_OUTER_BOUND('',#1426,.T.);
#1004=FACE_OUTER_BOUND('',#1427,.T.);
#1005=FACE_OUTER_BOUND('',#1440,.T.);
#1006=FACE_OUTER_BOUND('',#1441,.T.);
#1007=FACE_OUTER_BOUND('',#1443,.T.);
#1008=FACE_OUTER_BOUND('',#1444,.T.);
#1009=FACE_OUTER_BOUND('',#1445,.T.);
#1010=FACE_OUTER_BOUND('',#1446,.T.);
#1011=FACE_OUTER_BOUND('',#1447,.T.);
#1012=FACE_OUTER_BOUND('',#1448,.T.);
#1013=FACE_OUTER_BOUND('',#1450,.T.);
#1014=FACE_OUTER_BOUND('',#1451,.T.);
#1015=FACE_OUTER_BOUND('',#1453,.T.);
#1016=FACE_OUTER_BOUND('',#1454,.T.);
#1017=FACE_OUTER_BOUND('',#1456,.T.);
#1018=FACE_OUTER_BOUND('',#1457,.T.);
#1019=FACE_OUTER_BOUND('',#1459,.T.);
#1020=FACE_OUTER_BOUND('',#1460,.T.);
#1021=FACE_OUTER_BOUND('',#1462,.T.);
#1022=FACE_OUTER_BOUND('',#1463,.T.);
#1023=FACE_OUTER_BOUND('',#1465,.T.);
#1024=FACE_OUTER_BOUND('',#1466,.T.);
#1025=FACE_OUTER_BOUND('',#1468,.T.);
#1026=FACE_OUTER_BOUND('',#1469,.T.);
#1027=FACE_OUTER_BOUND('',#1471,.T.);
#1028=FACE_OUTER_BOUND('',#1472,.T.);
#1029=FACE_OUTER_BOUND('',#1473,.T.);
#1030=FACE_OUTER_BOUND('',#1474,.T.);
#1031=FACE_OUTER_BOUND('',#1475,.T.);
#1032=FACE_OUTER_BOUND('',#1476,.T.);
#1033=FACE_OUTER_BOUND('',#1477,.T.);
#1034=FACE_OUTER_BOUND('',#1478,.T.);
#1035=FACE_OUTER_BOUND('',#1479,.T.);
#1036=FACE_OUTER_BOUND('',#1480,.T.);
#1037=FACE_OUTER_BOUND('',#1482,.T.);
#1038=FACE_OUTER_BOUND('',#1483,.T.);
#1039=FACE_OUTER_BOUND('',#1485,.T.);
#1040=FACE_OUTER_BOUND('',#1486,.T.);
#1041=FACE_OUTER_BOUND('',#1488,.T.);
#1042=FACE_OUTER_BOUND('',#1489,.T.);
#1043=FACE_OUTER_BOUND('',#1491,.T.);
#1044=FACE_OUTER_BOUND('',#1492,.T.);
#1045=FACE_OUTER_BOUND('',#1494,.T.);
#1046=FACE_OUTER_BOUND('',#1495,.T.);
#1047=FACE_OUTER_BOUND('',#1497,.T.);
#1048=FACE_OUTER_BOUND('',#1498,.T.);
#1049=FACE_OUTER_BOUND('',#1500,.T.);
#1050=FACE_OUTER_BOUND('',#1501,.T.);
#1051=FACE_OUTER_BOUND('',#1503,.T.);
#1052=FACE_OUTER_BOUND('',#1504,.T.);
#1053=FACE_OUTER_BOUND('',#1505,.T.);
#1054=FACE_OUTER_BOUND('',#1506,.T.);
#1055=FACE_OUTER_BOUND('',#1507,.T.);
#1056=FACE_OUTER_BOUND('',#1508,.T.);
#1057=FACE_OUTER_BOUND('',#1509,.T.);
#1058=FACE_OUTER_BOUND('',#1511,.T.);
#1059=FACE_OUTER_BOUND('',#1512,.T.);
#1060=FACE_OUTER_BOUND('',#1513,.T.);
#1061=FACE_OUTER_BOUND('',#1514,.T.);
#1062=FACE_OUTER_BOUND('',#1515,.T.);
#1063=FACE_OUTER_BOUND('',#1516,.T.);
#1064=FACE_OUTER_BOUND('',#1518,.T.);
#1065=FACE_OUTER_BOUND('',#1519,.T.);
#1066=FACE_OUTER_BOUND('',#1520,.T.);
#1067=FACE_OUTER_BOUND('',#1521,.T.);
#1068=FACE_OUTER_BOUND('',#1522,.T.);
#1069=FACE_OUTER_BOUND('',#1523,.T.);
#1070=FACE_OUTER_BOUND('',#1525,.T.);
#1071=FACE_OUTER_BOUND('',#1526,.T.);
#1072=FACE_OUTER_BOUND('',#1527,.T.);
#1073=FACE_OUTER_BOUND('',#1528,.T.);
#1074=FACE_OUTER_BOUND('',#1529,.T.);
#1075=FACE_OUTER_BOUND('',#1530,.T.);
#1076=FACE_OUTER_BOUND('',#1531,.T.);
#1077=FACE_OUTER_BOUND('',#1532,.T.);
#1078=FACE_OUTER_BOUND('',#1533,.T.);
#1380=EDGE_LOOP('',(#5069,#5070,#5071,#5072));
#1381=EDGE_LOOP('',(#5073,#5074,#5075,#5076));
#1382=EDGE_LOOP('',(#5077,#5078,#5079,#5080));
#1383=EDGE_LOOP('',(#5081,#5082,#5083,#5084,#5085,#5086));
#1384=EDGE_LOOP('',(#5087,#5088,#5089,#5090,#5091));
#1385=EDGE_LOOP('',(#5092,#5093,#5094,#5095,#5096));
#1386=EDGE_LOOP('',(#5097,#5098,#5099,#5100));
#1387=EDGE_LOOP('',(#5101,#5102,#5103,#5104));
#1388=EDGE_LOOP('',(#5105,#5106,#5107,#5108,#5109,#5110));
#1389=EDGE_LOOP('',(#5111,#5112,#5113,#5114,#5115));
#1390=EDGE_LOOP('',(#5116,#5117,#5118,#5119,#5120));
#1391=EDGE_LOOP('',(#5121,#5122,#5123,#5124));
#1392=EDGE_LOOP('',(#5125,#5126,#5127,#5128,#5129,#5130));
#1393=EDGE_LOOP('',(#5131,#5132,#5133,#5134,#5135));
#1394=EDGE_LOOP('',(#5136,#5137,#5138,#5139,#5140));
#1395=EDGE_LOOP('',(#5141,#5142,#5143,#5144));
#1396=EDGE_LOOP('',(#5145,#5146,#5147,#5148));
#1397=EDGE_LOOP('',(#5149,#5150,#5151,#5152));
#1398=EDGE_LOOP('',(#5153));
#1399=EDGE_LOOP('',(#5154,#5155,#5156,#5157,#5158,#5159,#5160,#5161,#5162,
#5163,#5164,#5165));
#1400=EDGE_LOOP('',(#5166));
#1401=EDGE_LOOP('',(#5167,#5168,#5169,#5170,#5171,#5172,#5173,#5174,#5175,
#5176,#5177,#5178));
#1402=EDGE_LOOP('',(#5179,#5180,#5181,#5182));
#1403=EDGE_LOOP('',(#5183,#5184,#5185,#5186,#5187,#5188,#5189,#5190,#5191,
#5192,#5193,#5194));
#1404=EDGE_LOOP('',(#5195));
#1405=EDGE_LOOP('',(#5196,#5197,#5198,#5199,#5200,#5201,#5202,#5203,#5204,
#5205,#5206,#5207));
#1406=EDGE_LOOP('',(#5208));
#1407=EDGE_LOOP('',(#5209));
#1408=EDGE_LOOP('',(#5210,#5211,#5212,#5213,#5214,#5215,#5216,#5217));
#1409=EDGE_LOOP('',(#5218));
#1410=EDGE_LOOP('',(#5219));
#1411=EDGE_LOOP('',(#5220,#5221,#5222,#5223,#5224,#5225));
#1412=EDGE_LOOP('',(#5226));
#1413=EDGE_LOOP('',(#5227));
#1414=EDGE_LOOP('',(#5228,#5229,#5230,#5231,#5232,#5233));
#1415=EDGE_LOOP('',(#5234));
#1416=EDGE_LOOP('',(#5235));
#1417=EDGE_LOOP('',(#5236,#5237,#5238,#5239,#5240,#5241));
#1418=EDGE_LOOP('',(#5242));
#1419=EDGE_LOOP('',(#5243));
#1420=EDGE_LOOP('',(#5244,#5245,#5246,#5247));
#1421=EDGE_LOOP('',(#5248));
#1422=EDGE_LOOP('',(#5249));
#1423=EDGE_LOOP('',(#5250,#5251,#5252,#5253));
#1424=EDGE_LOOP('',(#5254));
#1425=EDGE_LOOP('',(#5255));
#1426=EDGE_LOOP('',(#5256,#5257,#5258,#5259));
#1427=EDGE_LOOP('',(#5260,#5261,#5262,#5263));
#1428=EDGE_LOOP('',(#5264,#5265));
#1429=EDGE_LOOP('',(#5266,#5267));
#1430=EDGE_LOOP('',(#5268,#5269));
#1431=EDGE_LOOP('',(#5270,#5271));
#1432=EDGE_LOOP('',(#5272,#5273));
#1433=EDGE_LOOP('',(#5274,#5275));
#1434=EDGE_LOOP('',(#5276,#5277));
#1435=EDGE_LOOP('',(#5278,#5279));
#1436=EDGE_LOOP('',(#5280,#5281));
#1437=EDGE_LOOP('',(#5282,#5283));
#1438=EDGE_LOOP('',(#5284,#5285));
#1439=EDGE_LOOP('',(#5286,#5287));
#1440=EDGE_LOOP('',(#5288));
#1441=EDGE_LOOP('',(#5289));
#1442=EDGE_LOOP('',(#5290));
#1443=EDGE_LOOP('',(#5291,#5292,#5293,#5294));
#1444=EDGE_LOOP('',(#5295,#5296,#5297,#5298,#5299));
#1445=EDGE_LOOP('',(#5300,#5301,#5302,#5303,#5304));
#1446=EDGE_LOOP('',(#5305,#5306,#5307,#5308,#5309));
#1447=EDGE_LOOP('',(#5310,#5311,#5312,#5313,#5314));
#1448=EDGE_LOOP('',(#5315));
#1449=EDGE_LOOP('',(#5316));
#1450=EDGE_LOOP('',(#5317,#5318,#5319,#5320,#5321,#5322,#5323,#5324));
#1451=EDGE_LOOP('',(#5325));
#1452=EDGE_LOOP('',(#5326));
#1453=EDGE_LOOP('',(#5327,#5328,#5329,#5330,#5331,#5332,#5333,#5334));
#1454=EDGE_LOOP('',(#5335));
#1455=EDGE_LOOP('',(#5336));
#1456=EDGE_LOOP('',(#5337,#5338,#5339,#5340,#5341,#5342));
#1457=EDGE_LOOP('',(#5343));
#1458=EDGE_LOOP('',(#5344));
#1459=EDGE_LOOP('',(#5345,#5346,#5347,#5348,#5349,#5350));
#1460=EDGE_LOOP('',(#5351));
#1461=EDGE_LOOP('',(#5352));
#1462=EDGE_LOOP('',(#5353,#5354,#5355,#5356,#5357,#5358));
#1463=EDGE_LOOP('',(#5359));
#1464=EDGE_LOOP('',(#5360));
#1465=EDGE_LOOP('',(#5361,#5362,#5363,#5364,#5365,#5366));
#1466=EDGE_LOOP('',(#5367));
#1467=EDGE_LOOP('',(#5368));
#1468=EDGE_LOOP('',(#5369,#5370,#5371,#5372,#5373,#5374));
#1469=EDGE_LOOP('',(#5375));
#1470=EDGE_LOOP('',(#5376));
#1471=EDGE_LOOP('',(#5377,#5378,#5379,#5380,#5381,#5382));
#1472=EDGE_LOOP('',(#5383,#5384,#5385,#5386,#5387));
#1473=EDGE_LOOP('',(#5388,#5389,#5390,#5391,#5392));
#1474=EDGE_LOOP('',(#5393,#5394,#5395,#5396,#5397));
#1475=EDGE_LOOP('',(#5398,#5399,#5400,#5401,#5402));
#1476=EDGE_LOOP('',(#5403,#5404,#5405,#5406,#5407));
#1477=EDGE_LOOP('',(#5408,#5409,#5410,#5411,#5412));
#1478=EDGE_LOOP('',(#5413,#5414,#5415,#5416,#5417));
#1479=EDGE_LOOP('',(#5418,#5419,#5420,#5421,#5422));
#1480=EDGE_LOOP('',(#5423));
#1481=EDGE_LOOP('',(#5424));
#1482=EDGE_LOOP('',(#5425,#5426,#5427,#5428));
#1483=EDGE_LOOP('',(#5429));
#1484=EDGE_LOOP('',(#5430));
#1485=EDGE_LOOP('',(#5431,#5432,#5433,#5434));
#1486=EDGE_LOOP('',(#5435));
#1487=EDGE_LOOP('',(#5436));
#1488=EDGE_LOOP('',(#5437,#5438,#5439,#5440));
#1489=EDGE_LOOP('',(#5441));
#1490=EDGE_LOOP('',(#5442));
#1491=EDGE_LOOP('',(#5443,#5444,#5445,#5446));
#1492=EDGE_LOOP('',(#5447));
#1493=EDGE_LOOP('',(#5448));
#1494=EDGE_LOOP('',(#5449,#5450,#5451,#5452));
#1495=EDGE_LOOP('',(#5453));
#1496=EDGE_LOOP('',(#5454));
#1497=EDGE_LOOP('',(#5455,#5456,#5457,#5458));
#1498=EDGE_LOOP('',(#5459));
#1499=EDGE_LOOP('',(#5460));
#1500=EDGE_LOOP('',(#5461,#5462,#5463,#5464));
#1501=EDGE_LOOP('',(#5465));
#1502=EDGE_LOOP('',(#5466));
#1503=EDGE_LOOP('',(#5467,#5468,#5469,#5470));
#1504=EDGE_LOOP('',(#5471,#5472,#5473,#5474));
#1505=EDGE_LOOP('',(#5475,#5476,#5477,#5478));
#1506=EDGE_LOOP('',(#5479,#5480,#5481,#5482,#5483,#5484,#5485));
#1507=EDGE_LOOP('',(#5486,#5487,#5488,#5489,#5490,#5491,#5492));
#1508=EDGE_LOOP('',(#5493,#5494,#5495,#5496));
#1509=EDGE_LOOP('',(#5497,#5498,#5499,#5500));
#1510=EDGE_LOOP('',(#5501,#5502,#5503,#5504));
#1511=EDGE_LOOP('',(#5505,#5506,#5507,#5508));
#1512=EDGE_LOOP('',(#5509,#5510,#5511,#5512));
#1513=EDGE_LOOP('',(#5513,#5514,#5515,#5516,#5517,#5518,#5519));
#1514=EDGE_LOOP('',(#5520,#5521,#5522,#5523,#5524,#5525,#5526));
#1515=EDGE_LOOP('',(#5527,#5528,#5529,#5530));
#1516=EDGE_LOOP('',(#5531,#5532,#5533,#5534));
#1517=EDGE_LOOP('',(#5535,#5536,#5537,#5538));
#1518=EDGE_LOOP('',(#5539,#5540,#5541,#5542));
#1519=EDGE_LOOP('',(#5543,#5544,#5545,#5546));
#1520=EDGE_LOOP('',(#5547,#5548,#5549,#5550,#5551,#5552,#5553));
#1521=EDGE_LOOP('',(#5554,#5555,#5556,#5557,#5558,#5559,#5560));
#1522=EDGE_LOOP('',(#5561,#5562,#5563,#5564));
#1523=EDGE_LOOP('',(#5565,#5566,#5567,#5568));
#1524=EDGE_LOOP('',(#5569,#5570,#5571,#5572));
#1525=EDGE_LOOP('',(#5573,#5574,#5575,#5576));
#1526=EDGE_LOOP('',(#5577,#5578,#5579,#5580));
#1527=EDGE_LOOP('',(#5581,#5582,#5583,#5584));
#1528=EDGE_LOOP('',(#5585,#5586,#5587,#5588));
#1529=EDGE_LOOP('',(#5589,#5590,#5591,#5592));
#1530=EDGE_LOOP('',(#5593,#5594,#5595,#5596));
#1531=EDGE_LOOP('',(#5597,#5598,#5599,#5600));
#1532=EDGE_LOOP('',(#5601,#5602,#5603,#5604));
#1533=EDGE_LOOP('',(#5605,#5606,#5607,#5608));
#1727=CIRCLE('',#6671,15.);
#1728=CIRCLE('',#6672,15.);
#1729=CIRCLE('',#6674,15.);
#1730=CIRCLE('',#6675,15.);
#1731=CIRCLE('',#6677,15.);
#1732=CIRCLE('',#6678,15.);
#1733=CIRCLE('',#6684,15.);
#1734=CIRCLE('',#6685,15.);
#1735=CIRCLE('',#6695,15.);
#1736=CIRCLE('',#6696,15.);
#1737=CIRCLE('',#6698,15.);
#1738=CIRCLE('',#6699,15.);
#1739=CIRCLE('',#6701,17.);
#1740=CIRCLE('',#6702,14.5);
#1741=CIRCLE('',#6703,14.5);
#1742=CIRCLE('',#6704,14.5);
#1743=CIRCLE('',#6706,17.);
#1744=CIRCLE('',#6709,12.9999999999984);
#1745=CIRCLE('',#6711,14.5);
#1746=CIRCLE('',#6712,14.5);
#1747=CIRCLE('',#6713,14.5);
#1748=CIRCLE('',#6715,4.00000000000012);
#1749=CIRCLE('',#6716,3.50000000000012);
#1750=CIRCLE('',#6719,4.00000000000001);
#1751=CIRCLE('',#6720,3.5);
#1752=CIRCLE('',#6723,4.00000000000001);
#1753=CIRCLE('',#6724,3.49999999999992);
#1754=CIRCLE('',#6727,4.);
#1755=CIRCLE('',#6728,3.49999999999998);
#1756=CIRCLE('',#6731,3.50000000000012);
#1757=CIRCLE('',#6732,2.80000000000012);
#1758=CIRCLE('',#6735,3.5);
#1759=CIRCLE('',#6736,2.79999999999998);
#1760=CIRCLE('',#6739,3.49999999999992);
#1761=CIRCLE('',#6740,2.79999999999991);
#1762=CIRCLE('',#6743,12.9999999999984);
#1763=CIRCLE('',#6746,3.49999999999998);
#1764=CIRCLE('',#6747,2.79999999999999);
#1765=CIRCLE('',#6754,4.00000000000012);
#1766=CIRCLE('',#6755,3.50000000000012);
#1767=CIRCLE('',#6758,4.00000000000012);
#1768=CIRCLE('',#6759,3.50000000000012);
#1769=CIRCLE('',#6762,4.00000000000001);
#1770=CIRCLE('',#6763,3.5);
#1771=CIRCLE('',#6766,4.00000000000001);
#1772=CIRCLE('',#6767,3.5);
#1773=CIRCLE('',#6770,4.00000000000001);
#1774=CIRCLE('',#6771,3.49999999999992);
#1775=CIRCLE('',#6774,4.00000000000001);
#1776=CIRCLE('',#6775,3.49999999999992);
#1777=CIRCLE('',#6778,4.);
#1778=CIRCLE('',#6779,3.49999999999998);
#1779=CIRCLE('',#6782,4.);
#1780=CIRCLE('',#6783,3.49999999999998);
#1781=CIRCLE('',#6786,2.80000000000012);
#1782=CIRCLE('',#6788,2.80000000000012);
#1783=CIRCLE('',#6790,2.79999999999998);
#1784=CIRCLE('',#6792,2.79999999999998);
#1785=CIRCLE('',#6794,2.79999999999991);
#1786=CIRCLE('',#6796,2.79999999999991);
#1787=CIRCLE('',#6798,2.79999999999999);
#1788=CIRCLE('',#6800,2.79999999999999);
#1789=CIRCLE('',#6802,3.50000000000012);
#1790=CIRCLE('',#6805,3.50000000000012);
#1791=CIRCLE('',#6808,3.5);
#1792=CIRCLE('',#6811,3.5);
#1793=CIRCLE('',#6814,3.49999999999992);
#1794=CIRCLE('',#6817,3.49999999999992);
#1795=CIRCLE('',#6820,3.49999999999998);
#1796=CIRCLE('',#6823,3.49999999999998);
#2054=LINE('',#12321,#2442);
#2055=LINE('',#12325,#2443);
#2056=LINE('',#12330,#2444);
#2057=LINE('',#12334,#2445);
#2058=LINE('',#12341,#2446);
#2059=LINE('',#12344,#2447);
#2060=LINE('',#12348,#2448);
#2061=LINE('',#12374,#2449);
#2062=LINE('',#12400,#2450);
#2063=LINE('',#12425,#2451);
#2064=LINE('',#12446,#2452);
#2065=LINE('',#12471,#2453);
#2066=LINE('',#12492,#2454);
#2067=LINE('',#12516,#2455);
#2068=LINE('',#12548,#2456);
#2069=LINE('',#12551,#2457);
#2070=LINE('',#12555,#2458);
#2071=LINE('',#12581,#2459);
#2072=LINE('',#12607,#2460);
#2073=LINE('',#12632,#2461);
#2074=LINE('',#12653,#2462);
#2075=LINE('',#12678,#2463);
#2076=LINE('',#12699,#2464);
#2077=LINE('',#12723,#2465);
#2078=LINE('',#12753,#2466);
#2079=LINE('',#12779,#2467);
#2080=LINE('',#12805,#2468);
#2081=LINE('',#12830,#2469);
#2082=LINE('',#12851,#2470);
#2083=LINE('',#12876,#2471);
#2084=LINE('',#12897,#2472);
#2085=LINE('',#12921,#2473);
#2086=LINE('',#12953,#2474);
#2087=LINE('',#12956,#2475);
#2088=LINE('',#12960,#2476);
#2089=LINE('',#12964,#2477);
#2090=LINE('',#12970,#2478);
#2091=LINE('',#12973,#2479);
#2092=LINE('',#12975,#2480);
#2093=LINE('',#12978,#2481);
#2094=LINE('',#12980,#2482);
#2095=LINE('',#12983,#2483);
#2096=LINE('',#12988,#2484);
#2097=LINE('',#12990,#2485);
#2098=LINE('',#12991,#2486);
#2099=LINE('',#12993,#2487);
#2100=LINE('',#12995,#2488);
#2101=LINE('',#12996,#2489);
#2102=LINE('',#12998,#2490);
#2103=LINE('',#13000,#2491);
#2104=LINE('',#13001,#2492);
#2105=LINE('',#13003,#2493);
#2106=LINE('',#13006,#2494);
#2107=LINE('',#13008,#2495);
#2108=LINE('',#13009,#2496);
#2109=LINE('',#13011,#2497);
#2110=LINE('',#13013,#2498);
#2111=LINE('',#13014,#2499);
#2112=LINE('',#13016,#2500);
#2113=LINE('',#13018,#2501);
#2114=LINE('',#13019,#2502);
#2115=LINE('',#13024,#2503);
#2116=LINE('',#13027,#2504);
#2117=LINE('',#13029,#2505);
#2118=LINE('',#13032,#2506);
#2119=LINE('',#13034,#2507);
#2120=LINE('',#13037,#2508);
#2121=LINE('',#13044,#2509);
#2122=LINE('',#13046,#2510);
#2123=LINE('',#13066,#2511);
#2124=LINE('',#13073,#2512);
#2125=LINE('',#13080,#2513);
#2126=LINE('',#13087,#2514);
#2127=LINE('',#13094,#2515);
#2128=LINE('',#13101,#2516);
#2129=LINE('',#13108,#2517);
#2130=LINE('',#13112,#2518);
#2131=LINE('',#13648,#2519);
#2132=LINE('',#13650,#2520);
#2133=LINE('',#13652,#2521);
#2134=LINE('',#13654,#2522);
#2135=LINE('',#13656,#2523);
#2136=LINE('',#13663,#2524);
#2137=LINE('',#13665,#2525);
#2138=LINE('',#13685,#2526);
#2139=LINE('',#13692,#2527);
#2140=LINE('',#13694,#2528);
#2141=LINE('',#13714,#2529);
#2142=LINE('',#13721,#2530);
#2143=LINE('',#13728,#2531);
#2144=LINE('',#13735,#2532);
#2145=LINE('',#13742,#2533);
#2146=LINE('',#13749,#2534);
#2147=LINE('',#13756,#2535);
#2148=LINE('',#13759,#2536);
#2149=LINE('',#13763,#2537);
#2150=LINE('',#13767,#2538);
#2151=LINE('',#13771,#2539);
#2152=LINE('',#13775,#2540);
#2153=LINE('',#13779,#2541);
#2154=LINE('',#13783,#2542);
#2155=LINE('',#13787,#2543);
#2156=LINE('',#13793,#2544);
#2157=LINE('',#13798,#2545);
#2158=LINE('',#13803,#2546);
#2159=LINE('',#13808,#2547);
#2160=LINE('',#13813,#2548);
#2161=LINE('',#13818,#2549);
#2162=LINE('',#13823,#2550);
#2163=LINE('',#13828,#2551);
#2164=LINE('',#13830,#2552);
#2165=LINE('',#13832,#2553);
#2166=LINE('',#13835,#2554);
#2167=LINE('',#13836,#2555);
#2168=LINE('',#13839,#2556);
#2169=LINE('',#13840,#2557);
#2170=LINE('',#13893,#2558);
#2171=LINE('',#13895,#2559);
#2172=LINE('',#13898,#2560);
#2173=LINE('',#13899,#2561);
#2174=LINE('',#13902,#2562);
#2175=LINE('',#13903,#2563);
#2176=LINE('',#13956,#2564);
#2177=LINE('',#13958,#2565);
#2178=LINE('',#13961,#2566);
#2179=LINE('',#13962,#2567);
#2180=LINE('',#13965,#2568);
#2181=LINE('',#13966,#2569);
#2182=LINE('',#14019,#2570);
#2183=LINE('',#14021,#2571);
#2184=LINE('',#14024,#2572);
#2185=LINE('',#14026,#2573);
#2186=LINE('',#14029,#2574);
#2187=LINE('',#14031,#2575);
#2442=VECTOR('',#7984,3.99999999999999);
#2443=VECTOR('',#7987,3.99999999999998);
#2444=VECTOR('',#7992,3.99999999999999);
#2445=VECTOR('',#7995,3.99999999999996);
#2446=VECTOR('',#8002,57.);
#2447=VECTOR('',#8005,57.);
#2448=VECTOR('',#8008,13.3544586520373);
#2449=VECTOR('',#8009,13.3544586520371);
#2450=VECTOR('',#8012,13.3319433271509);
#2451=VECTOR('',#8013,13.3319433271509);
#2452=VECTOR('',#8016,13.2704303156128);
#2453=VECTOR('',#8017,13.2704303156126);
#2454=VECTOR('',#8020,3.88631345570718);
#2455=VECTOR('',#8021,3.88631345570666);
#2456=VECTOR('',#8026,57.);
#2457=VECTOR('',#8029,57.);
#2458=VECTOR('',#8032,13.3544586520373);
#2459=VECTOR('',#8033,13.3544586520371);
#2460=VECTOR('',#8036,13.3319433271511);
#2461=VECTOR('',#8037,13.3319433271509);
#2462=VECTOR('',#8040,13.2704303156128);
#2463=VECTOR('',#8041,13.2704303156126);
#2464=VECTOR('',#8044,3.88631345570709);
#2465=VECTOR('',#8045,3.88631345570659);
#2466=VECTOR('',#8048,13.3544586520373);
#2467=VECTOR('',#8049,13.3544586520371);
#2468=VECTOR('',#8052,13.331943327151);
#2469=VECTOR('',#8053,13.3319433271509);
#2470=VECTOR('',#8056,13.2704303156128);
#2471=VECTOR('',#8057,13.2704303156126);
#2472=VECTOR('',#8060,3.88631345570711);
#2473=VECTOR('',#8061,3.8863134557066);
#2474=VECTOR('',#8066,57.);
#2475=VECTOR('',#8069,57.);
#2476=VECTOR('',#8072,3.99999999999998);
#2477=VECTOR('',#8075,3.99999999999998);
#2478=VECTOR('',#8082,0.561081020730737);
#2479=VECTOR('',#8085,0.561081020730727);
#2480=VECTOR('',#8086,0.561081020730758);
#2481=VECTOR('',#8089,0.561081020730749);
#2482=VECTOR('',#8090,0.561081020730754);
#2483=VECTOR('',#8093,0.561081020730736);
#2484=VECTOR('',#8098,0.999999999999974);
#2485=VECTOR('',#8099,1.00000000000001);
#2486=VECTOR('',#8100,0.999999999999884);
#2487=VECTOR('',#8101,1.);
#2488=VECTOR('',#8102,1.00000000000001);
#2489=VECTOR('',#8103,0.999999999999921);
#2490=VECTOR('',#8104,0.999999999999996);
#2491=VECTOR('',#8105,0.999999999999991);
#2492=VECTOR('',#8106,0.99999999999989);
#2493=VECTOR('',#8109,17.);
#2494=VECTOR('',#8112,0.999999999999894);
#2495=VECTOR('',#8113,1.00000000000001);
#2496=VECTOR('',#8114,0.999999999999984);
#2497=VECTOR('',#8115,0.99999999999989);
#2498=VECTOR('',#8116,0.999999999999991);
#2499=VECTOR('',#8117,0.999999999999996);
#2500=VECTOR('',#8118,0.999999999999925);
#2501=VECTOR('',#8119,1.00000000000001);
#2502=VECTOR('',#8120,1.00000000000002);
#2503=VECTOR('',#8125,0.56108102073074);
#2504=VECTOR('',#8128,0.561081020730741);
#2505=VECTOR('',#8129,0.561081020730736);
#2506=VECTOR('',#8132,0.561081020730754);
#2507=VECTOR('',#8133,0.561081020730749);
#2508=VECTOR('',#8136,0.561081020730719);
#2509=VECTOR('',#8145,4.00000000000012);
#2510=VECTOR('',#8146,0.519472430034522);
#2511=VECTOR('',#8147,0.519472430034611);
#2512=VECTOR('',#8156,4.00000000000001);
#2513=VECTOR('',#8165,4.00000000000001);
#2514=VECTOR('',#8174,4.);
#2515=VECTOR('',#8183,3.50000000000012);
#2516=VECTOR('',#8192,3.5);
#2517=VECTOR('',#8201,3.49999999999992);
#2518=VECTOR('',#8206,12.9999999999984);
#2519=VECTOR('',#8217,3.49999999999998);
#2520=VECTOR('',#8220,2.80000000000012);
#2521=VECTOR('',#8223,2.79999999999998);
#2522=VECTOR('',#8226,2.79999999999991);
#2523=VECTOR('',#8229,2.79999999999999);
#2524=VECTOR('',#8238,4.00000000000012);
#2525=VECTOR('',#8239,0.519472430034534);
#2526=VECTOR('',#8240,0.519472430034598);
#2527=VECTOR('',#8249,4.00000000000012);
#2528=VECTOR('',#8250,0.519472430034482);
#2529=VECTOR('',#8251,0.519472430034555);
#2530=VECTOR('',#8260,4.00000000000001);
#2531=VECTOR('',#8269,4.00000000000001);
#2532=VECTOR('',#8278,4.00000000000001);
#2533=VECTOR('',#8287,4.00000000000001);
#2534=VECTOR('',#8296,4.);
#2535=VECTOR('',#8305,4.);
#2536=VECTOR('',#8308,2.80000000000012);
#2537=VECTOR('',#8313,2.80000000000012);
#2538=VECTOR('',#8318,2.79999999999998);
#2539=VECTOR('',#8323,2.79999999999998);
#2540=VECTOR('',#8328,2.79999999999991);
#2541=VECTOR('',#8333,2.79999999999991);
#2542=VECTOR('',#8338,2.79999999999999);
#2543=VECTOR('',#8343,2.79999999999999);
#2544=VECTOR('',#8352,3.50000000000012);
#2545=VECTOR('',#8359,3.50000000000012);
#2546=VECTOR('',#8366,3.5);
#2547=VECTOR('',#8373,3.5);
#2548=VECTOR('',#8380,3.49999999999992);
#2549=VECTOR('',#8387,3.49999999999992);
#2550=VECTOR('',#8394,3.49999999999998);
#2551=VECTOR('',#8401,3.49999999999998);
#2552=VECTOR('',#8404,57.);
#2553=VECTOR('',#8407,57.);
#2554=VECTOR('',#8410,0.519472430034682);
#2555=VECTOR('',#8411,43.8431457505075);
#2556=VECTOR('',#8414,43.8431457505077);
#2557=VECTOR('',#8415,0.519472430034611);
#2558=VECTOR('',#8420,57.);
#2559=VECTOR('',#8423,57.);
#2560=VECTOR('',#8426,0.51947243003468);
#2561=VECTOR('',#8427,43.8431457505077);
#2562=VECTOR('',#8430,43.8431457505077);
#2563=VECTOR('',#8431,0.519472430034606);
#2564=VECTOR('',#8436,57.);
#2565=VECTOR('',#8439,57.);
#2566=VECTOR('',#8442,0.5194724300347);
#2567=VECTOR('',#8443,43.8431457505077);
#2568=VECTOR('',#8446,43.8431457505077);
#2569=VECTOR('',#8447,0.519472430034622);
#2570=VECTOR('',#8452,3.99999999999998);
#2571=VECTOR('',#8455,3.99999999999998);
#2572=VECTOR('',#8460,3.99999999999997);
#2573=VECTOR('',#8463,4.);
#2574=VECTOR('',#8468,3.99999999999998);
#2575=VECTOR('',#8471,3.99999999999998);
#2944=VERTEX_POINT('',#12319);
#2945=VERTEX_POINT('',#12320);
#2946=VERTEX_POINT('',#12322);
#2947=VERTEX_POINT('',#12324);
#2948=VERTEX_POINT('',#12328);
#2949=VERTEX_POINT('',#12329);
#2950=VERTEX_POINT('',#12331);
#2951=VERTEX_POINT('',#12333);
#2952=VERTEX_POINT('',#12337);
#2953=VERTEX_POINT('',#12338);
#2954=VERTEX_POINT('',#12340);
#2955=VERTEX_POINT('',#12342);
#2956=VERTEX_POINT('',#12346);
#2957=VERTEX_POINT('',#12347);
#2958=VERTEX_POINT('',#12349);
#2959=VERTEX_POINT('',#12358);
#2960=VERTEX_POINT('',#12373);
#2961=VERTEX_POINT('',#12375);
#2962=VERTEX_POINT('',#12399);
#2963=VERTEX_POINT('',#12401);
#2964=VERTEX_POINT('',#12410);
#2965=VERTEX_POINT('',#12445);
#2966=VERTEX_POINT('',#12447);
#2967=VERTEX_POINT('',#12458);
#2968=VERTEX_POINT('',#12491);
#2969=VERTEX_POINT('',#12515);
#2970=VERTEX_POINT('',#12544);
#2971=VERTEX_POINT('',#12545);
#2972=VERTEX_POINT('',#12547);
#2973=VERTEX_POINT('',#12549);
#2974=VERTEX_POINT('',#12553);
#2975=VERTEX_POINT('',#12554);
#2976=VERTEX_POINT('',#12556);
#2977=VERTEX_POINT('',#12565);
#2978=VERTEX_POINT('',#12580);
#2979=VERTEX_POINT('',#12582);
#2980=VERTEX_POINT('',#12606);
#2981=VERTEX_POINT('',#12608);
#2982=VERTEX_POINT('',#12617);
#2983=VERTEX_POINT('',#12652);
#2984=VERTEX_POINT('',#12654);
#2985=VERTEX_POINT('',#12663);
#2986=VERTEX_POINT('',#12698);
#2987=VERTEX_POINT('',#12722);
#2988=VERTEX_POINT('',#12751);
#2989=VERTEX_POINT('',#12752);
#2990=VERTEX_POINT('',#12754);
#2991=VERTEX_POINT('',#12763);
#2992=VERTEX_POINT('',#12778);
#2993=VERTEX_POINT('',#12780);
#2994=VERTEX_POINT('',#12804);
#2995=VERTEX_POINT('',#12806);
#2996=VERTEX_POINT('',#12815);
#2997=VERTEX_POINT('',#12850);
#2998=VERTEX_POINT('',#12852);
#2999=VERTEX_POINT('',#12863);
#3000=VERTEX_POINT('',#12896);
#3001=VERTEX_POINT('',#12920);
#3002=VERTEX_POINT('',#12949);
#3003=VERTEX_POINT('',#12950);
#3004=VERTEX_POINT('',#12952);
#3005=VERTEX_POINT('',#12954);
#3006=VERTEX_POINT('',#12958);
#3007=VERTEX_POINT('',#12959);
#3008=VERTEX_POINT('',#12961);
#3009=VERTEX_POINT('',#12963);
#3010=VERTEX_POINT('',#12967);
#3011=VERTEX_POINT('',#12969);
#3012=VERTEX_POINT('',#12971);
#3013=VERTEX_POINT('',#12974);
#3014=VERTEX_POINT('',#12976);
#3015=VERTEX_POINT('',#12979);
#3016=VERTEX_POINT('',#12981);
#3017=VERTEX_POINT('',#12985);
#3018=VERTEX_POINT('',#12987);
#3019=VERTEX_POINT('',#12989);
#3020=VERTEX_POINT('',#12992);
#3021=VERTEX_POINT('',#12994);
#3022=VERTEX_POINT('',#12997);
#3023=VERTEX_POINT('',#12999);
#3024=VERTEX_POINT('',#13005);
#3025=VERTEX_POINT('',#13007);
#3026=VERTEX_POINT('',#13010);
#3027=VERTEX_POINT('',#13012);
#3028=VERTEX_POINT('',#13015);
#3029=VERTEX_POINT('',#13017);
#3030=VERTEX_POINT('',#13020);
#3031=VERTEX_POINT('',#13023);
#3032=VERTEX_POINT('',#13025);
#3033=VERTEX_POINT('',#13028);
#3034=VERTEX_POINT('',#13030);
#3035=VERTEX_POINT('',#13033);
#3036=VERTEX_POINT('',#13035);
#3037=VERTEX_POINT('',#13039);
#3038=VERTEX_POINT('',#13041);
#3039=VERTEX_POINT('',#13045);
#3040=VERTEX_POINT('',#13047);
#3041=VERTEX_POINT('',#13068);
#3042=VERTEX_POINT('',#13070);
#3043=VERTEX_POINT('',#13075);
#3044=VERTEX_POINT('',#13077);
#3045=VERTEX_POINT('',#13082);
#3046=VERTEX_POINT('',#13084);
#3047=VERTEX_POINT('',#13089);
#3048=VERTEX_POINT('',#13091);
#3049=VERTEX_POINT('',#13096);
#3050=VERTEX_POINT('',#13098);
#3051=VERTEX_POINT('',#13103);
#3052=VERTEX_POINT('',#13105);
#3053=VERTEX_POINT('',#13110);
#3054=VERTEX_POINT('',#13113);
#3055=VERTEX_POINT('',#13114);
#3056=VERTEX_POINT('',#13160);
#3057=VERTEX_POINT('',#13161);
#3058=VERTEX_POINT('',#13207);
#3059=VERTEX_POINT('',#13208);
#3060=VERTEX_POINT('',#13250);
#3061=VERTEX_POINT('',#13251);
#3062=VERTEX_POINT('',#13293);
#3063=VERTEX_POINT('',#13294);
#3064=VERTEX_POINT('',#13336);
#3065=VERTEX_POINT('',#13337);
#3066=VERTEX_POINT('',#13379);
#3067=VERTEX_POINT('',#13380);
#3068=VERTEX_POINT('',#13422);
#3069=VERTEX_POINT('',#13423);
#3070=VERTEX_POINT('',#13465);
#3071=VERTEX_POINT('',#13466);
#3072=VERTEX_POINT('',#13512);
#3073=VERTEX_POINT('',#13513);
#3074=VERTEX_POINT('',#13555);
#3075=VERTEX_POINT('',#13556);
#3076=VERTEX_POINT('',#13598);
#3077=VERTEX_POINT('',#13599);
#3078=VERTEX_POINT('',#13643);
#3079=VERTEX_POINT('',#13645);
#3080=VERTEX_POINT('',#13658);
#3081=VERTEX_POINT('',#13660);
#3082=VERTEX_POINT('',#13664);
#3083=VERTEX_POINT('',#13666);
#3084=VERTEX_POINT('',#13687);
#3085=VERTEX_POINT('',#13689);
#3086=VERTEX_POINT('',#13693);
#3087=VERTEX_POINT('',#13695);
#3088=VERTEX_POINT('',#13716);
#3089=VERTEX_POINT('',#13718);
#3090=VERTEX_POINT('',#13723);
#3091=VERTEX_POINT('',#13725);
#3092=VERTEX_POINT('',#13730);
#3093=VERTEX_POINT('',#13732);
#3094=VERTEX_POINT('',#13737);
#3095=VERTEX_POINT('',#13739);
#3096=VERTEX_POINT('',#13744);
#3097=VERTEX_POINT('',#13746);
#3098=VERTEX_POINT('',#13751);
#3099=VERTEX_POINT('',#13753);
#3100=VERTEX_POINT('',#13758);
#3101=VERTEX_POINT('',#13762);
#3102=VERTEX_POINT('',#13766);
#3103=VERTEX_POINT('',#13770);
#3104=VERTEX_POINT('',#13774);
#3105=VERTEX_POINT('',#13778);
#3106=VERTEX_POINT('',#13782);
#3107=VERTEX_POINT('',#13786);
#3108=VERTEX_POINT('',#13790);
#3109=VERTEX_POINT('',#13795);
#3110=VERTEX_POINT('',#13800);
#3111=VERTEX_POINT('',#13805);
#3112=VERTEX_POINT('',#13810);
#3113=VERTEX_POINT('',#13815);
#3114=VERTEX_POINT('',#13820);
#3115=VERTEX_POINT('',#13825);
#3116=VERTEX_POINT('',#13834);
#3117=VERTEX_POINT('',#13838);
#3118=VERTEX_POINT('',#13897);
#3119=VERTEX_POINT('',#13901);
#3120=VERTEX_POINT('',#13960);
#3121=VERTEX_POINT('',#13964);
#3682=EDGE_CURVE('',#2944,#2945,#2054,.F.);
#3683=EDGE_CURVE('',#2946,#2944,#1727,.T.);
#3684=EDGE_CURVE('',#2947,#2946,#2055,.T.);
#3685=EDGE_CURVE('',#2947,#2945,#1728,.T.);
#3686=EDGE_CURVE('',#2948,#2949,#2056,.T.);
#3687=EDGE_CURVE('',#2948,#2950,#1729,.T.);
#3688=EDGE_CURVE('',#2951,#2950,#2057,.F.);
#3689=EDGE_CURVE('',#2949,#2951,#1730,.T.);
#3690=EDGE_CURVE('',#2952,#2953,#1731,.T.);
#3691=EDGE_CURVE('',#2953,#2954,#2058,.F.);
#3692=EDGE_CURVE('',#2955,#2954,#1732,.T.);
#3693=EDGE_CURVE('',#2955,#2952,#2059,.T.);
#3694=EDGE_CURVE('',#2956,#2957,#2060,.T.);
#3695=EDGE_CURVE('',#2958,#2956,#411,.T.);
#3696=EDGE_CURVE('',#2959,#2958,#412,.T.);
#3697=EDGE_CURVE('',#2960,#2959,#2061,.F.);
#3698=EDGE_CURVE('',#2961,#2960,#413,.T.);
#3699=EDGE_CURVE('',#2957,#2961,#414,.T.);
#3700=EDGE_CURVE('',#2962,#2956,#2062,.T.);
#3701=EDGE_CURVE('',#2963,#2962,#415,.T.);
#3702=EDGE_CURVE('',#2964,#2963,#416,.T.);
#3703=EDGE_CURVE('',#2959,#2964,#2063,.F.);
#3704=EDGE_CURVE('',#2956,#2959,#417,.T.);
#3705=EDGE_CURVE('',#2965,#2962,#2064,.T.);
#3706=EDGE_CURVE('',#2966,#2965,#418,.T.);
#3707=EDGE_CURVE('',#2967,#2966,#419,.T.);
#3708=EDGE_CURVE('',#2964,#2967,#2065,.F.);
#3709=EDGE_CURVE('',#2962,#2964,#420,.T.);
#3710=EDGE_CURVE('',#2967,#2968,#2066,.F.);
#3711=EDGE_CURVE('',#2965,#2967,#421,.T.);
#3712=EDGE_CURVE('',#2969,#2965,#2067,.T.);
#3713=EDGE_CURVE('',#2968,#2969,#422,.T.);
#3714=EDGE_CURVE('',#2970,#2971,#1733,.T.);
#3715=EDGE_CURVE('',#2971,#2972,#2068,.F.);
#3716=EDGE_CURVE('',#2973,#2972,#1734,.T.);
#3717=EDGE_CURVE('',#2973,#2970,#2069,.T.);
#3718=EDGE_CURVE('',#2974,#2975,#2070,.T.);
#3719=EDGE_CURVE('',#2976,#2974,#423,.T.);
#3720=EDGE_CURVE('',#2977,#2976,#424,.T.);
#3721=EDGE_CURVE('',#2978,#2977,#2071,.F.);
#3722=EDGE_CURVE('',#2979,#2978,#425,.T.);
#3723=EDGE_CURVE('',#2975,#2979,#426,.T.);
#3724=EDGE_CURVE('',#2980,#2974,#2072,.T.);
#3725=EDGE_CURVE('',#2981,#2980,#427,.T.);
#3726=EDGE_CURVE('',#2982,#2981,#428,.T.);
#3727=EDGE_CURVE('',#2977,#2982,#2073,.F.);
#3728=EDGE_CURVE('',#2974,#2977,#429,.T.);
#3729=EDGE_CURVE('',#2983,#2980,#2074,.T.);
#3730=EDGE_CURVE('',#2984,#2983,#430,.T.);
#3731=EDGE_CURVE('',#2985,#2984,#431,.T.);
#3732=EDGE_CURVE('',#2982,#2985,#2075,.F.);
#3733=EDGE_CURVE('',#2980,#2982,#432,.T.);
#3734=EDGE_CURVE('',#2985,#2986,#2076,.F.);
#3735=EDGE_CURVE('',#2983,#2985,#433,.T.);
#3736=EDGE_CURVE('',#2987,#2983,#2077,.T.);
#3737=EDGE_CURVE('',#2986,#2987,#434,.T.);
#3738=EDGE_CURVE('',#2988,#2989,#2078,.T.);
#3739=EDGE_CURVE('',#2990,#2988,#435,.T.);
#3740=EDGE_CURVE('',#2991,#2990,#436,.T.);
#3741=EDGE_CURVE('',#2992,#2991,#2079,.F.);
#3742=EDGE_CURVE('',#2993,#2992,#437,.T.);
#3743=EDGE_CURVE('',#2989,#2993,#438,.T.);
#3744=EDGE_CURVE('',#2994,#2988,#2080,.T.);
#3745=EDGE_CURVE('',#2995,#2994,#439,.T.);
#3746=EDGE_CURVE('',#2996,#2995,#440,.T.);
#3747=EDGE_CURVE('',#2991,#2996,#2081,.F.);
#3748=EDGE_CURVE('',#2988,#2991,#441,.T.);
#3749=EDGE_CURVE('',#2997,#2994,#2082,.T.);
#3750=EDGE_CURVE('',#2998,#2997,#442,.T.);
#3751=EDGE_CURVE('',#2999,#2998,#443,.T.);
#3752=EDGE_CURVE('',#2996,#2999,#2083,.F.);
#3753=EDGE_CURVE('',#2994,#2996,#444,.T.);
#3754=EDGE_CURVE('',#2999,#3000,#2084,.F.);
#3755=EDGE_CURVE('',#2997,#2999,#445,.T.);
#3756=EDGE_CURVE('',#3001,#2997,#2085,.T.);
#3757=EDGE_CURVE('',#3000,#3001,#446,.T.);
#3758=EDGE_CURVE('',#3002,#3003,#1735,.T.);
#3759=EDGE_CURVE('',#3002,#3004,#2086,.T.);
#3760=EDGE_CURVE('',#3004,#3005,#1736,.T.);
#3761=EDGE_CURVE('',#3005,#3003,#2087,.F.);
#3762=EDGE_CURVE('',#3006,#3007,#2088,.T.);
#3763=EDGE_CURVE('',#3006,#3008,#1737,.T.);
#3764=EDGE_CURVE('',#3009,#3008,#2089,.F.);
#3765=EDGE_CURVE('',#3007,#3009,#1738,.T.);
#3766=EDGE_CURVE('',#3010,#3010,#1739,.T.);
#3767=EDGE_CURVE('',#3011,#3004,#2090,.T.);
#3768=EDGE_CURVE('',#3012,#3011,#1740,.F.);
#3769=EDGE_CURVE('',#3012,#2953,#2091,.T.);
#3770=EDGE_CURVE('',#3013,#2952,#2092,.T.);
#3771=EDGE_CURVE('',#3014,#3013,#1741,.F.);
#3772=EDGE_CURVE('',#3014,#2971,#2093,.T.);
#3773=EDGE_CURVE('',#3015,#2970,#2094,.T.);
#3774=EDGE_CURVE('',#3016,#3015,#1742,.F.);
#3775=EDGE_CURVE('',#3016,#3005,#2095,.T.);
#3776=EDGE_CURVE('',#3017,#3017,#1743,.T.);
#3777=EDGE_CURVE('',#3018,#2944,#2096,.T.);
#3778=EDGE_CURVE('',#3019,#3018,#2097,.T.);
#3779=EDGE_CURVE('',#2949,#3019,#2098,.T.);
#3780=EDGE_CURVE('',#3020,#2951,#2099,.T.);
#3781=EDGE_CURVE('',#3021,#3020,#2100,.T.);
#3782=EDGE_CURVE('',#3007,#3021,#2101,.T.);
#3783=EDGE_CURVE('',#3022,#3009,#2102,.T.);
#3784=EDGE_CURVE('',#3023,#3022,#2103,.T.);
#3785=EDGE_CURVE('',#2946,#3023,#2104,.T.);
#3786=EDGE_CURVE('',#3017,#3010,#2105,.T.);
#3787=EDGE_CURVE('',#2948,#3024,#2106,.T.);
#3788=EDGE_CURVE('',#3024,#3025,#2107,.T.);
#3789=EDGE_CURVE('',#3025,#2945,#2108,.T.);
#3790=EDGE_CURVE('',#2947,#3026,#2109,.T.);
#3791=EDGE_CURVE('',#3026,#3027,#2110,.T.);
#3792=EDGE_CURVE('',#3027,#3008,#2111,.T.);
#3793=EDGE_CURVE('',#3006,#3028,#2112,.T.);
#3794=EDGE_CURVE('',#3028,#3029,#2113,.T.);
#3795=EDGE_CURVE('',#3029,#2950,#2114,.T.);
#3796=EDGE_CURVE('',#3030,#3030,#1744,.T.);
#3797=EDGE_CURVE('',#3031,#2954,#2115,.T.);
#3798=EDGE_CURVE('',#3032,#3031,#1745,.F.);
#3799=EDGE_CURVE('',#3002,#3032,#2116,.T.);
#3800=EDGE_CURVE('',#3033,#3003,#2117,.T.);
#3801=EDGE_CURVE('',#3034,#3033,#1746,.F.);
#3802=EDGE_CURVE('',#2973,#3034,#2118,.T.);
#3803=EDGE_CURVE('',#3035,#2972,#2119,.T.);
#3804=EDGE_CURVE('',#3036,#3035,#1747,.F.);
#3805=EDGE_CURVE('',#2955,#3036,#2120,.T.);
#3806=EDGE_CURVE('',#3037,#3037,#1748,.T.);
#3807=EDGE_CURVE('',#3038,#3038,#1749,.T.);
#3808=EDGE_CURVE('',#3037,#2993,#2121,.T.);
#3809=EDGE_CURVE('',#3039,#2992,#2122,.T.);
#3810=EDGE_CURVE('',#3039,#3040,#447,.T.);
#3811=EDGE_CURVE('',#3040,#2989,#2123,.T.);
#3812=EDGE_CURVE('',#3041,#3041,#1750,.T.);
#3813=EDGE_CURVE('',#3042,#3042,#1751,.T.);
#3814=EDGE_CURVE('',#3041,#2990,#2124,.T.);
#3815=EDGE_CURVE('',#3043,#3043,#1752,.T.);
#3816=EDGE_CURVE('',#3044,#3044,#1753,.T.);
#3817=EDGE_CURVE('',#3043,#2995,#2125,.T.);
#3818=EDGE_CURVE('',#3045,#3045,#1754,.T.);
#3819=EDGE_CURVE('',#3046,#3046,#1755,.T.);
#3820=EDGE_CURVE('',#3045,#2998,#2126,.T.);
#3821=EDGE_CURVE('',#3047,#3047,#1756,.T.);
#3822=EDGE_CURVE('',#3048,#3048,#1757,.T.);
#3823=EDGE_CURVE('',#3047,#3038,#2127,.T.);
#3824=EDGE_CURVE('',#3049,#3049,#1758,.T.);
#3825=EDGE_CURVE('',#3050,#3050,#1759,.T.);
#3826=EDGE_CURVE('',#3049,#3042,#2128,.T.);
#3827=EDGE_CURVE('',#3051,#3051,#1760,.T.);
#3828=EDGE_CURVE('',#3052,#3052,#1761,.T.);
#3829=EDGE_CURVE('',#3051,#3044,#2129,.T.);
#3830=EDGE_CURVE('',#3053,#3053,#1762,.F.);
#3831=EDGE_CURVE('',#3053,#3030,#2130,.T.);
#3832=EDGE_CURVE('',#3054,#3055,#448,.T.);
#3833=EDGE_CURVE('',#3055,#3054,#449,.T.);
#3834=EDGE_CURVE('',#3056,#3057,#450,.T.);
#3835=EDGE_CURVE('',#3057,#3056,#451,.T.);
#3836=EDGE_CURVE('',#3058,#3059,#452,.T.);
#3837=EDGE_CURVE('',#3059,#3058,#453,.T.);
#3838=EDGE_CURVE('',#3060,#3061,#454,.T.);
#3839=EDGE_CURVE('',#3061,#3060,#455,.T.);
#3840=EDGE_CURVE('',#3062,#3063,#456,.T.);
#3841=EDGE_CURVE('',#3063,#3062,#457,.T.);
#3842=EDGE_CURVE('',#3064,#3065,#458,.T.);
#3843=EDGE_CURVE('',#3065,#3064,#459,.T.);
#3844=EDGE_CURVE('',#3066,#3067,#460,.T.);
#3845=EDGE_CURVE('',#3067,#3066,#461,.T.);
#3846=EDGE_CURVE('',#3068,#3069,#462,.T.);
#3847=EDGE_CURVE('',#3069,#3068,#463,.T.);
#3848=EDGE_CURVE('',#3070,#3071,#464,.T.);
#3849=EDGE_CURVE('',#3071,#3070,#465,.T.);
#3850=EDGE_CURVE('',#3072,#3073,#466,.T.);
#3851=EDGE_CURVE('',#3073,#3072,#467,.T.);
#3852=EDGE_CURVE('',#3074,#3075,#468,.T.);
#3853=EDGE_CURVE('',#3075,#3074,#469,.T.);
#3854=EDGE_CURVE('',#3076,#3077,#470,.T.);
#3855=EDGE_CURVE('',#3077,#3076,#471,.T.);
#3856=EDGE_CURVE('',#3078,#3078,#1763,.T.);
#3857=EDGE_CURVE('',#3079,#3079,#1764,.T.);
#3858=EDGE_CURVE('',#3078,#3046,#2131,.T.);
#3859=EDGE_CURVE('',#3077,#3048,#2132,.T.);
#3860=EDGE_CURVE('',#3075,#3050,#2133,.T.);
#3861=EDGE_CURVE('',#3073,#3052,#2134,.T.);
#3862=EDGE_CURVE('',#3071,#3079,#2135,.T.);
#3863=EDGE_CURVE('',#3080,#3080,#1765,.T.);
#3864=EDGE_CURVE('',#3081,#3081,#1766,.T.);
#3865=EDGE_CURVE('',#3080,#2961,#2136,.T.);
#3866=EDGE_CURVE('',#3082,#2960,#2137,.T.);
#3867=EDGE_CURVE('',#3082,#3083,#472,.T.);
#3868=EDGE_CURVE('',#3083,#2957,#2138,.T.);
#3869=EDGE_CURVE('',#3084,#3084,#1767,.T.);
#3870=EDGE_CURVE('',#3085,#3085,#1768,.T.);
#3871=EDGE_CURVE('',#3084,#2979,#2139,.T.);
#3872=EDGE_CURVE('',#3086,#2978,#2140,.T.);
#3873=EDGE_CURVE('',#3086,#3087,#473,.T.);
#3874=EDGE_CURVE('',#3087,#2975,#2141,.T.);
#3875=EDGE_CURVE('',#3088,#3088,#1769,.T.);
#3876=EDGE_CURVE('',#3089,#3089,#1770,.T.);
#3877=EDGE_CURVE('',#3088,#2958,#2142,.T.);
#3878=EDGE_CURVE('',#3090,#3090,#1771,.T.);
#3879=EDGE_CURVE('',#3091,#3091,#1772,.T.);
#3880=EDGE_CURVE('',#3090,#2976,#2143,.T.);
#3881=EDGE_CURVE('',#3092,#3092,#1773,.T.);
#3882=EDGE_CURVE('',#3093,#3093,#1774,.T.);
#3883=EDGE_CURVE('',#3092,#2963,#2144,.T.);
#3884=EDGE_CURVE('',#3094,#3094,#1775,.T.);
#3885=EDGE_CURVE('',#3095,#3095,#1776,.T.);
#3886=EDGE_CURVE('',#3094,#2981,#2145,.T.);
#3887=EDGE_CURVE('',#3096,#3096,#1777,.T.);
#3888=EDGE_CURVE('',#3097,#3097,#1778,.T.);
#3889=EDGE_CURVE('',#3096,#2966,#2146,.T.);
#3890=EDGE_CURVE('',#3098,#3098,#1779,.T.);
#3891=EDGE_CURVE('',#3099,#3099,#1780,.T.);
#3892=EDGE_CURVE('',#3098,#2984,#2147,.T.);
#3893=EDGE_CURVE('',#3069,#3100,#2148,.T.);
#3894=EDGE_CURVE('',#3100,#3100,#1781,.F.);
#3895=EDGE_CURVE('',#3067,#3101,#2149,.T.);
#3896=EDGE_CURVE('',#3101,#3101,#1782,.F.);
#3897=EDGE_CURVE('',#3065,#3102,#2150,.T.);
#3898=EDGE_CURVE('',#3102,#3102,#1783,.F.);
#3899=EDGE_CURVE('',#3063,#3103,#2151,.T.);
#3900=EDGE_CURVE('',#3103,#3103,#1784,.F.);
#3901=EDGE_CURVE('',#3061,#3104,#2152,.T.);
#3902=EDGE_CURVE('',#3104,#3104,#1785,.F.);
#3903=EDGE_CURVE('',#3059,#3105,#2153,.T.);
#3904=EDGE_CURVE('',#3105,#3105,#1786,.F.);
#3905=EDGE_CURVE('',#3057,#3106,#2154,.T.);
#3906=EDGE_CURVE('',#3106,#3106,#1787,.F.);
#3907=EDGE_CURVE('',#3055,#3107,#2155,.T.);
#3908=EDGE_CURVE('',#3107,#3107,#1788,.F.);
#3909=EDGE_CURVE('',#3108,#3108,#1789,.T.);
#3910=EDGE_CURVE('',#3108,#3081,#2156,.T.);
#3911=EDGE_CURVE('',#3109,#3109,#1790,.T.);
#3912=EDGE_CURVE('',#3109,#3085,#2157,.T.);
#3913=EDGE_CURVE('',#3110,#3110,#1791,.T.);
#3914=EDGE_CURVE('',#3110,#3089,#2158,.T.);
#3915=EDGE_CURVE('',#3111,#3111,#1792,.T.);
#3916=EDGE_CURVE('',#3111,#3091,#2159,.T.);
#3917=EDGE_CURVE('',#3112,#3112,#1793,.T.);
#3918=EDGE_CURVE('',#3112,#3093,#2160,.T.);
#3919=EDGE_CURVE('',#3113,#3113,#1794,.T.);
#3920=EDGE_CURVE('',#3113,#3095,#2161,.T.);
#3921=EDGE_CURVE('',#3114,#3114,#1795,.T.);
#3922=EDGE_CURVE('',#3114,#3097,#2162,.T.);
#3923=EDGE_CURVE('',#3115,#3115,#1796,.T.);
#3924=EDGE_CURVE('',#3115,#3099,#2163,.T.);
#3925=EDGE_CURVE('',#3033,#3016,#2164,.T.);
#3926=EDGE_CURVE('',#3015,#3034,#2165,.F.);
#3927=EDGE_CURVE('',#3116,#3000,#2166,.T.);
#3928=EDGE_CURVE('',#3116,#3039,#2167,.T.);
#3929=EDGE_CURVE('',#3040,#3117,#2168,.F.);
#3930=EDGE_CURVE('',#3117,#3001,#2169,.T.);
#3931=EDGE_CURVE('',#3117,#3116,#474,.T.);
#3932=EDGE_CURVE('',#3035,#3014,#2170,.T.);
#3933=EDGE_CURVE('',#3013,#3036,#2171,.F.);
#3934=EDGE_CURVE('',#3118,#2986,#2172,.T.);
#3935=EDGE_CURVE('',#3118,#3086,#2173,.T.);
#3936=EDGE_CURVE('',#3087,#3119,#2174,.F.);
#3937=EDGE_CURVE('',#3119,#2987,#2175,.T.);
#3938=EDGE_CURVE('',#3119,#3118,#475,.T.);
#3939=EDGE_CURVE('',#3031,#3012,#2176,.T.);
#3940=EDGE_CURVE('',#3011,#3032,#2177,.F.);
#3941=EDGE_CURVE('',#3120,#2968,#2178,.T.);
#3942=EDGE_CURVE('',#3120,#3082,#2179,.T.);
#3943=EDGE_CURVE('',#3083,#3121,#2180,.F.);
#3944=EDGE_CURVE('',#3121,#2969,#2181,.T.);
#3945=EDGE_CURVE('',#3121,#3120,#476,.T.);
#3946=EDGE_CURVE('',#3027,#3022,#2182,.T.);
#3947=EDGE_CURVE('',#3026,#3023,#2183,.T.);
#3948=EDGE_CURVE('',#3029,#3020,#2184,.T.);
#3949=EDGE_CURVE('',#3028,#3021,#2185,.T.);
#3950=EDGE_CURVE('',#3025,#3018,#2186,.T.);
#3951=EDGE_CURVE('',#3024,#3019,#2187,.T.);
#5069=ORIENTED_EDGE('',*,*,#3682,.F.);
#5070=ORIENTED_EDGE('',*,*,#3683,.F.);
#5071=ORIENTED_EDGE('',*,*,#3684,.F.);
#5072=ORIENTED_EDGE('',*,*,#3685,.T.);
#5073=ORIENTED_EDGE('',*,*,#3686,.F.);
#5074=ORIENTED_EDGE('',*,*,#3687,.T.);
#5075=ORIENTED_EDGE('',*,*,#3688,.F.);
#5076=ORIENTED_EDGE('',*,*,#3689,.F.);
#5077=ORIENTED_EDGE('',*,*,#3690,.T.);
#5078=ORIENTED_EDGE('',*,*,#3691,.T.);
#5079=ORIENTED_EDGE('',*,*,#3692,.F.);
#5080=ORIENTED_EDGE('',*,*,#3693,.T.);
#5081=ORIENTED_EDGE('',*,*,#3694,.F.);
#5082=ORIENTED_EDGE('',*,*,#3695,.F.);
#5083=ORIENTED_EDGE('',*,*,#3696,.F.);
#5084=ORIENTED_EDGE('',*,*,#3697,.F.);
#5085=ORIENTED_EDGE('',*,*,#3698,.F.);
#5086=ORIENTED_EDGE('',*,*,#3699,.F.);
#5087=ORIENTED_EDGE('',*,*,#3700,.F.);
#5088=ORIENTED_EDGE('',*,*,#3701,.F.);
#5089=ORIENTED_EDGE('',*,*,#3702,.F.);
#5090=ORIENTED_EDGE('',*,*,#3703,.F.);
#5091=ORIENTED_EDGE('',*,*,#3704,.F.);
#5092=ORIENTED_EDGE('',*,*,#3705,.F.);
#5093=ORIENTED_EDGE('',*,*,#3706,.F.);
#5094=ORIENTED_EDGE('',*,*,#3707,.F.);
#5095=ORIENTED_EDGE('',*,*,#3708,.F.);
#5096=ORIENTED_EDGE('',*,*,#3709,.F.);
#5097=ORIENTED_EDGE('',*,*,#3710,.F.);
#5098=ORIENTED_EDGE('',*,*,#3711,.F.);
#5099=ORIENTED_EDGE('',*,*,#3712,.F.);
#5100=ORIENTED_EDGE('',*,*,#3713,.F.);
#5101=ORIENTED_EDGE('',*,*,#3714,.T.);
#5102=ORIENTED_EDGE('',*,*,#3715,.T.);
#5103=ORIENTED_EDGE('',*,*,#3716,.F.);
#5104=ORIENTED_EDGE('',*,*,#3717,.T.);
#5105=ORIENTED_EDGE('',*,*,#3718,.F.);
#5106=ORIENTED_EDGE('',*,*,#3719,.F.);
#5107=ORIENTED_EDGE('',*,*,#3720,.F.);
#5108=ORIENTED_EDGE('',*,*,#3721,.F.);
#5109=ORIENTED_EDGE('',*,*,#3722,.F.);
#5110=ORIENTED_EDGE('',*,*,#3723,.F.);
#5111=ORIENTED_EDGE('',*,*,#3724,.F.);
#5112=ORIENTED_EDGE('',*,*,#3725,.F.);
#5113=ORIENTED_EDGE('',*,*,#3726,.F.);
#5114=ORIENTED_EDGE('',*,*,#3727,.F.);
#5115=ORIENTED_EDGE('',*,*,#3728,.F.);
#5116=ORIENTED_EDGE('',*,*,#3729,.F.);
#5117=ORIENTED_EDGE('',*,*,#3730,.F.);
#5118=ORIENTED_EDGE('',*,*,#3731,.F.);
#5119=ORIENTED_EDGE('',*,*,#3732,.F.);
#5120=ORIENTED_EDGE('',*,*,#3733,.F.);
#5121=ORIENTED_EDGE('',*,*,#3734,.F.);
#5122=ORIENTED_EDGE('',*,*,#3735,.F.);
#5123=ORIENTED_EDGE('',*,*,#3736,.F.);
#5124=ORIENTED_EDGE('',*,*,#3737,.F.);
#5125=ORIENTED_EDGE('',*,*,#3738,.F.);
#5126=ORIENTED_EDGE('',*,*,#3739,.F.);
#5127=ORIENTED_EDGE('',*,*,#3740,.F.);
#5128=ORIENTED_EDGE('',*,*,#3741,.F.);
#5129=ORIENTED_EDGE('',*,*,#3742,.F.);
#5130=ORIENTED_EDGE('',*,*,#3743,.F.);
#5131=ORIENTED_EDGE('',*,*,#3744,.F.);
#5132=ORIENTED_EDGE('',*,*,#3745,.F.);
#5133=ORIENTED_EDGE('',*,*,#3746,.F.);
#5134=ORIENTED_EDGE('',*,*,#3747,.F.);
#5135=ORIENTED_EDGE('',*,*,#3748,.F.);
#5136=ORIENTED_EDGE('',*,*,#3749,.F.);
#5137=ORIENTED_EDGE('',*,*,#3750,.F.);
#5138=ORIENTED_EDGE('',*,*,#3751,.F.);
#5139=ORIENTED_EDGE('',*,*,#3752,.F.);
#5140=ORIENTED_EDGE('',*,*,#3753,.F.);
#5141=ORIENTED_EDGE('',*,*,#3754,.F.);
#5142=ORIENTED_EDGE('',*,*,#3755,.F.);
#5143=ORIENTED_EDGE('',*,*,#3756,.F.);
#5144=ORIENTED_EDGE('',*,*,#3757,.F.);
#5145=ORIENTED_EDGE('',*,*,#3758,.F.);
#5146=ORIENTED_EDGE('',*,*,#3759,.T.);
#5147=ORIENTED_EDGE('',*,*,#3760,.T.);
#5148=ORIENTED_EDGE('',*,*,#3761,.T.);
#5149=ORIENTED_EDGE('',*,*,#3762,.F.);
#5150=ORIENTED_EDGE('',*,*,#3763,.T.);
#5151=ORIENTED_EDGE('',*,*,#3764,.F.);
#5152=ORIENTED_EDGE('',*,*,#3765,.F.);
#5153=ORIENTED_EDGE('',*,*,#3766,.T.);
#5154=ORIENTED_EDGE('',*,*,#3760,.F.);
#5155=ORIENTED_EDGE('',*,*,#3767,.F.);
#5156=ORIENTED_EDGE('',*,*,#3768,.F.);
#5157=ORIENTED_EDGE('',*,*,#3769,.T.);
#5158=ORIENTED_EDGE('',*,*,#3690,.F.);
#5159=ORIENTED_EDGE('',*,*,#3770,.F.);
#5160=ORIENTED_EDGE('',*,*,#3771,.F.);
#5161=ORIENTED_EDGE('',*,*,#3772,.T.);
#5162=ORIENTED_EDGE('',*,*,#3714,.F.);
#5163=ORIENTED_EDGE('',*,*,#3773,.F.);
#5164=ORIENTED_EDGE('',*,*,#3774,.F.);
#5165=ORIENTED_EDGE('',*,*,#3775,.T.);
#5166=ORIENTED_EDGE('',*,*,#3776,.F.);
#5167=ORIENTED_EDGE('',*,*,#3683,.T.);
#5168=ORIENTED_EDGE('',*,*,#3777,.F.);
#5169=ORIENTED_EDGE('',*,*,#3778,.F.);
#5170=ORIENTED_EDGE('',*,*,#3779,.F.);
#5171=ORIENTED_EDGE('',*,*,#3689,.T.);
#5172=ORIENTED_EDGE('',*,*,#3780,.F.);
#5173=ORIENTED_EDGE('',*,*,#3781,.F.);
#5174=ORIENTED_EDGE('',*,*,#3782,.F.);
#5175=ORIENTED_EDGE('',*,*,#3765,.T.);
#5176=ORIENTED_EDGE('',*,*,#3783,.F.);
#5177=ORIENTED_EDGE('',*,*,#3784,.F.);
#5178=ORIENTED_EDGE('',*,*,#3785,.F.);
#5179=ORIENTED_EDGE('',*,*,#3776,.T.);
#5180=ORIENTED_EDGE('',*,*,#3786,.T.);
#5181=ORIENTED_EDGE('',*,*,#3766,.F.);
#5182=ORIENTED_EDGE('',*,*,#3786,.F.);
#5183=ORIENTED_EDGE('',*,*,#3687,.F.);
#5184=ORIENTED_EDGE('',*,*,#3787,.T.);
#5185=ORIENTED_EDGE('',*,*,#3788,.T.);
#5186=ORIENTED_EDGE('',*,*,#3789,.T.);
#5187=ORIENTED_EDGE('',*,*,#3685,.F.);
#5188=ORIENTED_EDGE('',*,*,#3790,.T.);
#5189=ORIENTED_EDGE('',*,*,#3791,.T.);
#5190=ORIENTED_EDGE('',*,*,#3792,.T.);
#5191=ORIENTED_EDGE('',*,*,#3763,.F.);
#5192=ORIENTED_EDGE('',*,*,#3793,.T.);
#5193=ORIENTED_EDGE('',*,*,#3794,.T.);
#5194=ORIENTED_EDGE('',*,*,#3795,.T.);
#5195=ORIENTED_EDGE('',*,*,#3796,.F.);
#5196=ORIENTED_EDGE('',*,*,#3797,.F.);
#5197=ORIENTED_EDGE('',*,*,#3798,.F.);
#5198=ORIENTED_EDGE('',*,*,#3799,.F.);
#5199=ORIENTED_EDGE('',*,*,#3758,.T.);
#5200=ORIENTED_EDGE('',*,*,#3800,.F.);
#5201=ORIENTED_EDGE('',*,*,#3801,.F.);
#5202=ORIENTED_EDGE('',*,*,#3802,.F.);
#5203=ORIENTED_EDGE('',*,*,#3716,.T.);
#5204=ORIENTED_EDGE('',*,*,#3803,.F.);
#5205=ORIENTED_EDGE('',*,*,#3804,.F.);
#5206=ORIENTED_EDGE('',*,*,#3805,.F.);
#5207=ORIENTED_EDGE('',*,*,#3692,.T.);
#5208=ORIENTED_EDGE('',*,*,#3806,.F.);
#5209=ORIENTED_EDGE('',*,*,#3807,.F.);
#5210=ORIENTED_EDGE('',*,*,#3806,.T.);
#5211=ORIENTED_EDGE('',*,*,#3808,.T.);
#5212=ORIENTED_EDGE('',*,*,#3742,.T.);
#5213=ORIENTED_EDGE('',*,*,#3809,.F.);
#5214=ORIENTED_EDGE('',*,*,#3810,.T.);
#5215=ORIENTED_EDGE('',*,*,#3811,.T.);
#5216=ORIENTED_EDGE('',*,*,#3743,.T.);
#5217=ORIENTED_EDGE('',*,*,#3808,.F.);
#5218=ORIENTED_EDGE('',*,*,#3812,.F.);
#5219=ORIENTED_EDGE('',*,*,#3813,.F.);
#5220=ORIENTED_EDGE('',*,*,#3812,.T.);
#5221=ORIENTED_EDGE('',*,*,#3814,.T.);
#5222=ORIENTED_EDGE('',*,*,#3739,.T.);
#5223=ORIENTED_EDGE('',*,*,#3748,.T.);
#5224=ORIENTED_EDGE('',*,*,#3740,.T.);
#5225=ORIENTED_EDGE('',*,*,#3814,.F.);
#5226=ORIENTED_EDGE('',*,*,#3815,.F.);
#5227=ORIENTED_EDGE('',*,*,#3816,.F.);
#5228=ORIENTED_EDGE('',*,*,#3815,.T.);
#5229=ORIENTED_EDGE('',*,*,#3817,.T.);
#5230=ORIENTED_EDGE('',*,*,#3745,.T.);
#5231=ORIENTED_EDGE('',*,*,#3753,.T.);
#5232=ORIENTED_EDGE('',*,*,#3746,.T.);
#5233=ORIENTED_EDGE('',*,*,#3817,.F.);
#5234=ORIENTED_EDGE('',*,*,#3818,.F.);
#5235=ORIENTED_EDGE('',*,*,#3819,.F.);
#5236=ORIENTED_EDGE('',*,*,#3818,.T.);
#5237=ORIENTED_EDGE('',*,*,#3820,.T.);
#5238=ORIENTED_EDGE('',*,*,#3750,.T.);
#5239=ORIENTED_EDGE('',*,*,#3755,.T.);
#5240=ORIENTED_EDGE('',*,*,#3751,.T.);
#5241=ORIENTED_EDGE('',*,*,#3820,.F.);
#5242=ORIENTED_EDGE('',*,*,#3821,.T.);
#5243=ORIENTED_EDGE('',*,*,#3822,.F.);
#5244=ORIENTED_EDGE('',*,*,#3821,.F.);
#5245=ORIENTED_EDGE('',*,*,#3823,.T.);
#5246=ORIENTED_EDGE('',*,*,#3807,.T.);
#5247=ORIENTED_EDGE('',*,*,#3823,.F.);
#5248=ORIENTED_EDGE('',*,*,#3824,.T.);
#5249=ORIENTED_EDGE('',*,*,#3825,.F.);
#5250=ORIENTED_EDGE('',*,*,#3824,.F.);
#5251=ORIENTED_EDGE('',*,*,#3826,.T.);
#5252=ORIENTED_EDGE('',*,*,#3813,.T.);
#5253=ORIENTED_EDGE('',*,*,#3826,.F.);
#5254=ORIENTED_EDGE('',*,*,#3827,.T.);
#5255=ORIENTED_EDGE('',*,*,#3828,.F.);
#5256=ORIENTED_EDGE('',*,*,#3827,.F.);
#5257=ORIENTED_EDGE('',*,*,#3829,.T.);
#5258=ORIENTED_EDGE('',*,*,#3816,.T.);
#5259=ORIENTED_EDGE('',*,*,#3829,.F.);
#5260=ORIENTED_EDGE('',*,*,#3830,.F.);
#5261=ORIENTED_EDGE('',*,*,#3831,.T.);
#5262=ORIENTED_EDGE('',*,*,#3796,.T.);
#5263=ORIENTED_EDGE('',*,*,#3831,.F.);
#5264=ORIENTED_EDGE('',*,*,#3832,.T.);
#5265=ORIENTED_EDGE('',*,*,#3833,.T.);
#5266=ORIENTED_EDGE('',*,*,#3834,.T.);
#5267=ORIENTED_EDGE('',*,*,#3835,.T.);
#5268=ORIENTED_EDGE('',*,*,#3836,.T.);
#5269=ORIENTED_EDGE('',*,*,#3837,.T.);
#5270=ORIENTED_EDGE('',*,*,#3838,.T.);
#5271=ORIENTED_EDGE('',*,*,#3839,.T.);
#5272=ORIENTED_EDGE('',*,*,#3840,.T.);
#5273=ORIENTED_EDGE('',*,*,#3841,.T.);
#5274=ORIENTED_EDGE('',*,*,#3842,.T.);
#5275=ORIENTED_EDGE('',*,*,#3843,.T.);
#5276=ORIENTED_EDGE('',*,*,#3844,.T.);
#5277=ORIENTED_EDGE('',*,*,#3845,.T.);
#5278=ORIENTED_EDGE('',*,*,#3846,.T.);
#5279=ORIENTED_EDGE('',*,*,#3847,.T.);
#5280=ORIENTED_EDGE('',*,*,#3848,.T.);
#5281=ORIENTED_EDGE('',*,*,#3849,.T.);
#5282=ORIENTED_EDGE('',*,*,#3850,.T.);
#5283=ORIENTED_EDGE('',*,*,#3851,.T.);
#5284=ORIENTED_EDGE('',*,*,#3852,.T.);
#5285=ORIENTED_EDGE('',*,*,#3853,.T.);
#5286=ORIENTED_EDGE('',*,*,#3854,.T.);
#5287=ORIENTED_EDGE('',*,*,#3855,.T.);
#5288=ORIENTED_EDGE('',*,*,#3830,.T.);
#5289=ORIENTED_EDGE('',*,*,#3856,.T.);
#5290=ORIENTED_EDGE('',*,*,#3857,.F.);
#5291=ORIENTED_EDGE('',*,*,#3856,.F.);
#5292=ORIENTED_EDGE('',*,*,#3858,.T.);
#5293=ORIENTED_EDGE('',*,*,#3819,.T.);
#5294=ORIENTED_EDGE('',*,*,#3858,.F.);
#5295=ORIENTED_EDGE('',*,*,#3854,.F.);
#5296=ORIENTED_EDGE('',*,*,#3855,.F.);
#5297=ORIENTED_EDGE('',*,*,#3859,.T.);
#5298=ORIENTED_EDGE('',*,*,#3822,.T.);
#5299=ORIENTED_EDGE('',*,*,#3859,.F.);
#5300=ORIENTED_EDGE('',*,*,#3852,.F.);
#5301=ORIENTED_EDGE('',*,*,#3853,.F.);
#5302=ORIENTED_EDGE('',*,*,#3860,.T.);
#5303=ORIENTED_EDGE('',*,*,#3825,.T.);
#5304=ORIENTED_EDGE('',*,*,#3860,.F.);
#5305=ORIENTED_EDGE('',*,*,#3850,.F.);
#5306=ORIENTED_EDGE('',*,*,#3851,.F.);
#5307=ORIENTED_EDGE('',*,*,#3861,.T.);
#5308=ORIENTED_EDGE('',*,*,#3828,.T.);
#5309=ORIENTED_EDGE('',*,*,#3861,.F.);
#5310=ORIENTED_EDGE('',*,*,#3848,.F.);
#5311=ORIENTED_EDGE('',*,*,#3849,.F.);
#5312=ORIENTED_EDGE('',*,*,#3862,.T.);
#5313=ORIENTED_EDGE('',*,*,#3857,.T.);
#5314=ORIENTED_EDGE('',*,*,#3862,.F.);
#5315=ORIENTED_EDGE('',*,*,#3863,.F.);
#5316=ORIENTED_EDGE('',*,*,#3864,.F.);
#5317=ORIENTED_EDGE('',*,*,#3863,.T.);
#5318=ORIENTED_EDGE('',*,*,#3865,.T.);
#5319=ORIENTED_EDGE('',*,*,#3698,.T.);
#5320=ORIENTED_EDGE('',*,*,#3866,.F.);
#5321=ORIENTED_EDGE('',*,*,#3867,.T.);
#5322=ORIENTED_EDGE('',*,*,#3868,.T.);
#5323=ORIENTED_EDGE('',*,*,#3699,.T.);
#5324=ORIENTED_EDGE('',*,*,#3865,.F.);
#5325=ORIENTED_EDGE('',*,*,#3869,.F.);
#5326=ORIENTED_EDGE('',*,*,#3870,.F.);
#5327=ORIENTED_EDGE('',*,*,#3869,.T.);
#5328=ORIENTED_EDGE('',*,*,#3871,.T.);
#5329=ORIENTED_EDGE('',*,*,#3722,.T.);
#5330=ORIENTED_EDGE('',*,*,#3872,.F.);
#5331=ORIENTED_EDGE('',*,*,#3873,.T.);
#5332=ORIENTED_EDGE('',*,*,#3874,.T.);
#5333=ORIENTED_EDGE('',*,*,#3723,.T.);
#5334=ORIENTED_EDGE('',*,*,#3871,.F.);
#5335=ORIENTED_EDGE('',*,*,#3875,.F.);
#5336=ORIENTED_EDGE('',*,*,#3876,.F.);
#5337=ORIENTED_EDGE('',*,*,#3875,.T.);
#5338=ORIENTED_EDGE('',*,*,#3877,.T.);
#5339=ORIENTED_EDGE('',*,*,#3695,.T.);
#5340=ORIENTED_EDGE('',*,*,#3704,.T.);
#5341=ORIENTED_EDGE('',*,*,#3696,.T.);
#5342=ORIENTED_EDGE('',*,*,#3877,.F.);
#5343=ORIENTED_EDGE('',*,*,#3878,.F.);
#5344=ORIENTED_EDGE('',*,*,#3879,.F.);
#5345=ORIENTED_EDGE('',*,*,#3878,.T.);
#5346=ORIENTED_EDGE('',*,*,#3880,.T.);
#5347=ORIENTED_EDGE('',*,*,#3719,.T.);
#5348=ORIENTED_EDGE('',*,*,#3728,.T.);
#5349=ORIENTED_EDGE('',*,*,#3720,.T.);
#5350=ORIENTED_EDGE('',*,*,#3880,.F.);
#5351=ORIENTED_EDGE('',*,*,#3881,.F.);
#5352=ORIENTED_EDGE('',*,*,#3882,.F.);
#5353=ORIENTED_EDGE('',*,*,#3881,.T.);
#5354=ORIENTED_EDGE('',*,*,#3883,.T.);
#5355=ORIENTED_EDGE('',*,*,#3701,.T.);
#5356=ORIENTED_EDGE('',*,*,#3709,.T.);
#5357=ORIENTED_EDGE('',*,*,#3702,.T.);
#5358=ORIENTED_EDGE('',*,*,#3883,.F.);
#5359=ORIENTED_EDGE('',*,*,#3884,.F.);
#5360=ORIENTED_EDGE('',*,*,#3885,.F.);
#5361=ORIENTED_EDGE('',*,*,#3884,.T.);
#5362=ORIENTED_EDGE('',*,*,#3886,.T.);
#5363=ORIENTED_EDGE('',*,*,#3725,.T.);
#5364=ORIENTED_EDGE('',*,*,#3733,.T.);
#5365=ORIENTED_EDGE('',*,*,#3726,.T.);
#5366=ORIENTED_EDGE('',*,*,#3886,.F.);
#5367=ORIENTED_EDGE('',*,*,#3887,.F.);
#5368=ORIENTED_EDGE('',*,*,#3888,.F.);
#5369=ORIENTED_EDGE('',*,*,#3887,.T.);
#5370=ORIENTED_EDGE('',*,*,#3889,.T.);
#5371=ORIENTED_EDGE('',*,*,#3706,.T.);
#5372=ORIENTED_EDGE('',*,*,#3711,.T.);
#5373=ORIENTED_EDGE('',*,*,#3707,.T.);
#5374=ORIENTED_EDGE('',*,*,#3889,.F.);
#5375=ORIENTED_EDGE('',*,*,#3890,.F.);
#5376=ORIENTED_EDGE('',*,*,#3891,.F.);
#5377=ORIENTED_EDGE('',*,*,#3890,.T.);
#5378=ORIENTED_EDGE('',*,*,#3892,.T.);
#5379=ORIENTED_EDGE('',*,*,#3730,.T.);
#5380=ORIENTED_EDGE('',*,*,#3735,.T.);
#5381=ORIENTED_EDGE('',*,*,#3731,.T.);
#5382=ORIENTED_EDGE('',*,*,#3892,.F.);
#5383=ORIENTED_EDGE('',*,*,#3846,.F.);
#5384=ORIENTED_EDGE('',*,*,#3847,.F.);
#5385=ORIENTED_EDGE('',*,*,#3893,.T.);
#5386=ORIENTED_EDGE('',*,*,#3894,.F.);
#5387=ORIENTED_EDGE('',*,*,#3893,.F.);
#5388=ORIENTED_EDGE('',*,*,#3844,.F.);
#5389=ORIENTED_EDGE('',*,*,#3845,.F.);
#5390=ORIENTED_EDGE('',*,*,#3895,.T.);
#5391=ORIENTED_EDGE('',*,*,#3896,.F.);
#5392=ORIENTED_EDGE('',*,*,#3895,.F.);
#5393=ORIENTED_EDGE('',*,*,#3842,.F.);
#5394=ORIENTED_EDGE('',*,*,#3843,.F.);
#5395=ORIENTED_EDGE('',*,*,#3897,.T.);
#5396=ORIENTED_EDGE('',*,*,#3898,.F.);
#5397=ORIENTED_EDGE('',*,*,#3897,.F.);
#5398=ORIENTED_EDGE('',*,*,#3840,.F.);
#5399=ORIENTED_EDGE('',*,*,#3841,.F.);
#5400=ORIENTED_EDGE('',*,*,#3899,.T.);
#5401=ORIENTED_EDGE('',*,*,#3900,.F.);
#5402=ORIENTED_EDGE('',*,*,#3899,.F.);
#5403=ORIENTED_EDGE('',*,*,#3838,.F.);
#5404=ORIENTED_EDGE('',*,*,#3839,.F.);
#5405=ORIENTED_EDGE('',*,*,#3901,.T.);
#5406=ORIENTED_EDGE('',*,*,#3902,.F.);
#5407=ORIENTED_EDGE('',*,*,#3901,.F.);
#5408=ORIENTED_EDGE('',*,*,#3836,.F.);
#5409=ORIENTED_EDGE('',*,*,#3837,.F.);
#5410=ORIENTED_EDGE('',*,*,#3903,.T.);
#5411=ORIENTED_EDGE('',*,*,#3904,.F.);
#5412=ORIENTED_EDGE('',*,*,#3903,.F.);
#5413=ORIENTED_EDGE('',*,*,#3834,.F.);
#5414=ORIENTED_EDGE('',*,*,#3835,.F.);
#5415=ORIENTED_EDGE('',*,*,#3905,.T.);
#5416=ORIENTED_EDGE('',*,*,#3906,.F.);
#5417=ORIENTED_EDGE('',*,*,#3905,.F.);
#5418=ORIENTED_EDGE('',*,*,#3832,.F.);
#5419=ORIENTED_EDGE('',*,*,#3833,.F.);
#5420=ORIENTED_EDGE('',*,*,#3907,.T.);
#5421=ORIENTED_EDGE('',*,*,#3908,.F.);
#5422=ORIENTED_EDGE('',*,*,#3907,.F.);
#5423=ORIENTED_EDGE('',*,*,#3909,.T.);
#5424=ORIENTED_EDGE('',*,*,#3896,.T.);
#5425=ORIENTED_EDGE('',*,*,#3909,.F.);
#5426=ORIENTED_EDGE('',*,*,#3910,.T.);
#5427=ORIENTED_EDGE('',*,*,#3864,.T.);
#5428=ORIENTED_EDGE('',*,*,#3910,.F.);
#5429=ORIENTED_EDGE('',*,*,#3911,.T.);
#5430=ORIENTED_EDGE('',*,*,#3894,.T.);
#5431=ORIENTED_EDGE('',*,*,#3911,.F.);
#5432=ORIENTED_EDGE('',*,*,#3912,.T.);
#5433=ORIENTED_EDGE('',*,*,#3870,.T.);
#5434=ORIENTED_EDGE('',*,*,#3912,.F.);
#5435=ORIENTED_EDGE('',*,*,#3913,.T.);
#5436=ORIENTED_EDGE('',*,*,#3900,.T.);
#5437=ORIENTED_EDGE('',*,*,#3913,.F.);
#5438=ORIENTED_EDGE('',*,*,#3914,.T.);
#5439=ORIENTED_EDGE('',*,*,#3876,.T.);
#5440=ORIENTED_EDGE('',*,*,#3914,.F.);
#5441=ORIENTED_EDGE('',*,*,#3915,.T.);
#5442=ORIENTED_EDGE('',*,*,#3898,.T.);
#5443=ORIENTED_EDGE('',*,*,#3915,.F.);
#5444=ORIENTED_EDGE('',*,*,#3916,.T.);
#5445=ORIENTED_EDGE('',*,*,#3879,.T.);
#5446=ORIENTED_EDGE('',*,*,#3916,.F.);
#5447=ORIENTED_EDGE('',*,*,#3917,.T.);
#5448=ORIENTED_EDGE('',*,*,#3904,.T.);
#5449=ORIENTED_EDGE('',*,*,#3917,.F.);
#5450=ORIENTED_EDGE('',*,*,#3918,.T.);
#5451=ORIENTED_EDGE('',*,*,#3882,.T.);
#5452=ORIENTED_EDGE('',*,*,#3918,.F.);
#5453=ORIENTED_EDGE('',*,*,#3919,.T.);
#5454=ORIENTED_EDGE('',*,*,#3902,.T.);
#5455=ORIENTED_EDGE('',*,*,#3919,.F.);
#5456=ORIENTED_EDGE('',*,*,#3920,.T.);
#5457=ORIENTED_EDGE('',*,*,#3885,.T.);
#5458=ORIENTED_EDGE('',*,*,#3920,.F.);
#5459=ORIENTED_EDGE('',*,*,#3921,.T.);
#5460=ORIENTED_EDGE('',*,*,#3908,.T.);
#5461=ORIENTED_EDGE('',*,*,#3921,.F.);
#5462=ORIENTED_EDGE('',*,*,#3922,.T.);
#5463=ORIENTED_EDGE('',*,*,#3888,.T.);
#5464=ORIENTED_EDGE('',*,*,#3922,.F.);
#5465=ORIENTED_EDGE('',*,*,#3923,.T.);
#5466=ORIENTED_EDGE('',*,*,#3906,.T.);
#5467=ORIENTED_EDGE('',*,*,#3923,.F.);
#5468=ORIENTED_EDGE('',*,*,#3924,.T.);
#5469=ORIENTED_EDGE('',*,*,#3891,.T.);
#5470=ORIENTED_EDGE('',*,*,#3924,.F.);
#5471=ORIENTED_EDGE('',*,*,#3775,.F.);
#5472=ORIENTED_EDGE('',*,*,#3925,.F.);
#5473=ORIENTED_EDGE('',*,*,#3800,.T.);
#5474=ORIENTED_EDGE('',*,*,#3761,.F.);
#5475=ORIENTED_EDGE('',*,*,#3802,.T.);
#5476=ORIENTED_EDGE('',*,*,#3926,.F.);
#5477=ORIENTED_EDGE('',*,*,#3773,.T.);
#5478=ORIENTED_EDGE('',*,*,#3717,.F.);
#5479=ORIENTED_EDGE('',*,*,#3741,.T.);
#5480=ORIENTED_EDGE('',*,*,#3747,.T.);
#5481=ORIENTED_EDGE('',*,*,#3752,.T.);
#5482=ORIENTED_EDGE('',*,*,#3754,.T.);
#5483=ORIENTED_EDGE('',*,*,#3927,.F.);
#5484=ORIENTED_EDGE('',*,*,#3928,.T.);
#5485=ORIENTED_EDGE('',*,*,#3809,.T.);
#5486=ORIENTED_EDGE('',*,*,#3756,.T.);
#5487=ORIENTED_EDGE('',*,*,#3749,.T.);
#5488=ORIENTED_EDGE('',*,*,#3744,.T.);
#5489=ORIENTED_EDGE('',*,*,#3738,.T.);
#5490=ORIENTED_EDGE('',*,*,#3811,.F.);
#5491=ORIENTED_EDGE('',*,*,#3929,.T.);
#5492=ORIENTED_EDGE('',*,*,#3930,.T.);
#5493=ORIENTED_EDGE('',*,*,#3757,.T.);
#5494=ORIENTED_EDGE('',*,*,#3930,.F.);
#5495=ORIENTED_EDGE('',*,*,#3931,.T.);
#5496=ORIENTED_EDGE('',*,*,#3927,.T.);
#5497=ORIENTED_EDGE('',*,*,#3801,.T.);
#5498=ORIENTED_EDGE('',*,*,#3925,.T.);
#5499=ORIENTED_EDGE('',*,*,#3774,.T.);
#5500=ORIENTED_EDGE('',*,*,#3926,.T.);
#5501=ORIENTED_EDGE('',*,*,#3929,.F.);
#5502=ORIENTED_EDGE('',*,*,#3810,.F.);
#5503=ORIENTED_EDGE('',*,*,#3928,.F.);
#5504=ORIENTED_EDGE('',*,*,#3931,.F.);
#5505=ORIENTED_EDGE('',*,*,#3772,.F.);
#5506=ORIENTED_EDGE('',*,*,#3932,.F.);
#5507=ORIENTED_EDGE('',*,*,#3803,.T.);
#5508=ORIENTED_EDGE('',*,*,#3715,.F.);
#5509=ORIENTED_EDGE('',*,*,#3805,.T.);
#5510=ORIENTED_EDGE('',*,*,#3933,.F.);
#5511=ORIENTED_EDGE('',*,*,#3770,.T.);
#5512=ORIENTED_EDGE('',*,*,#3693,.F.);
#5513=ORIENTED_EDGE('',*,*,#3721,.T.);
#5514=ORIENTED_EDGE('',*,*,#3727,.T.);
#5515=ORIENTED_EDGE('',*,*,#3732,.T.);
#5516=ORIENTED_EDGE('',*,*,#3734,.T.);
#5517=ORIENTED_EDGE('',*,*,#3934,.F.);
#5518=ORIENTED_EDGE('',*,*,#3935,.T.);
#5519=ORIENTED_EDGE('',*,*,#3872,.T.);
#5520=ORIENTED_EDGE('',*,*,#3736,.T.);
#5521=ORIENTED_EDGE('',*,*,#3729,.T.);
#5522=ORIENTED_EDGE('',*,*,#3724,.T.);
#5523=ORIENTED_EDGE('',*,*,#3718,.T.);
#5524=ORIENTED_EDGE('',*,*,#3874,.F.);
#5525=ORIENTED_EDGE('',*,*,#3936,.T.);
#5526=ORIENTED_EDGE('',*,*,#3937,.T.);
#5527=ORIENTED_EDGE('',*,*,#3737,.T.);
#5528=ORIENTED_EDGE('',*,*,#3937,.F.);
#5529=ORIENTED_EDGE('',*,*,#3938,.T.);
#5530=ORIENTED_EDGE('',*,*,#3934,.T.);
#5531=ORIENTED_EDGE('',*,*,#3804,.T.);
#5532=ORIENTED_EDGE('',*,*,#3932,.T.);
#5533=ORIENTED_EDGE('',*,*,#3771,.T.);
#5534=ORIENTED_EDGE('',*,*,#3933,.T.);
#5535=ORIENTED_EDGE('',*,*,#3936,.F.);
#5536=ORIENTED_EDGE('',*,*,#3873,.F.);
#5537=ORIENTED_EDGE('',*,*,#3935,.F.);
#5538=ORIENTED_EDGE('',*,*,#3938,.F.);
#5539=ORIENTED_EDGE('',*,*,#3769,.F.);
#5540=ORIENTED_EDGE('',*,*,#3939,.F.);
#5541=ORIENTED_EDGE('',*,*,#3797,.T.);
#5542=ORIENTED_EDGE('',*,*,#3691,.F.);
#5543=ORIENTED_EDGE('',*,*,#3799,.T.);
#5544=ORIENTED_EDGE('',*,*,#3940,.F.);
#5545=ORIENTED_EDGE('',*,*,#3767,.T.);
#5546=ORIENTED_EDGE('',*,*,#3759,.F.);
#5547=ORIENTED_EDGE('',*,*,#3697,.T.);
#5548=ORIENTED_EDGE('',*,*,#3703,.T.);
#5549=ORIENTED_EDGE('',*,*,#3708,.T.);
#5550=ORIENTED_EDGE('',*,*,#3710,.T.);
#5551=ORIENTED_EDGE('',*,*,#3941,.F.);
#5552=ORIENTED_EDGE('',*,*,#3942,.T.);
#5553=ORIENTED_EDGE('',*,*,#3866,.T.);
#5554=ORIENTED_EDGE('',*,*,#3712,.T.);
#5555=ORIENTED_EDGE('',*,*,#3705,.T.);
#5556=ORIENTED_EDGE('',*,*,#3700,.T.);
#5557=ORIENTED_EDGE('',*,*,#3694,.T.);
#5558=ORIENTED_EDGE('',*,*,#3868,.F.);
#5559=ORIENTED_EDGE('',*,*,#3943,.T.);
#5560=ORIENTED_EDGE('',*,*,#3944,.T.);
#5561=ORIENTED_EDGE('',*,*,#3713,.T.);
#5562=ORIENTED_EDGE('',*,*,#3944,.F.);
#5563=ORIENTED_EDGE('',*,*,#3945,.T.);
#5564=ORIENTED_EDGE('',*,*,#3941,.T.);
#5565=ORIENTED_EDGE('',*,*,#3798,.T.);
#5566=ORIENTED_EDGE('',*,*,#3939,.T.);
#5567=ORIENTED_EDGE('',*,*,#3768,.T.);
#5568=ORIENTED_EDGE('',*,*,#3940,.T.);
#5569=ORIENTED_EDGE('',*,*,#3943,.F.);
#5570=ORIENTED_EDGE('',*,*,#3867,.F.);
#5571=ORIENTED_EDGE('',*,*,#3942,.F.);
#5572=ORIENTED_EDGE('',*,*,#3945,.F.);
#5573=ORIENTED_EDGE('',*,*,#3764,.T.);
#5574=ORIENTED_EDGE('',*,*,#3792,.F.);
#5575=ORIENTED_EDGE('',*,*,#3946,.T.);
#5576=ORIENTED_EDGE('',*,*,#3783,.T.);
#5577=ORIENTED_EDGE('',*,*,#3684,.T.);
#5578=ORIENTED_EDGE('',*,*,#3785,.T.);
#5579=ORIENTED_EDGE('',*,*,#3947,.F.);
#5580=ORIENTED_EDGE('',*,*,#3790,.F.);
#5581=ORIENTED_EDGE('',*,*,#3947,.T.);
#5582=ORIENTED_EDGE('',*,*,#3784,.T.);
#5583=ORIENTED_EDGE('',*,*,#3946,.F.);
#5584=ORIENTED_EDGE('',*,*,#3791,.F.);
#5585=ORIENTED_EDGE('',*,*,#3688,.T.);
#5586=ORIENTED_EDGE('',*,*,#3795,.F.);
#5587=ORIENTED_EDGE('',*,*,#3948,.T.);
#5588=ORIENTED_EDGE('',*,*,#3780,.T.);
#5589=ORIENTED_EDGE('',*,*,#3762,.T.);
#5590=ORIENTED_EDGE('',*,*,#3782,.T.);
#5591=ORIENTED_EDGE('',*,*,#3949,.F.);
#5592=ORIENTED_EDGE('',*,*,#3793,.F.);
#5593=ORIENTED_EDGE('',*,*,#3949,.T.);
#5594=ORIENTED_EDGE('',*,*,#3781,.T.);
#5595=ORIENTED_EDGE('',*,*,#3948,.F.);
#5596=ORIENTED_EDGE('',*,*,#3794,.F.);
#5597=ORIENTED_EDGE('',*,*,#3682,.T.);
#5598=ORIENTED_EDGE('',*,*,#3789,.F.);
#5599=ORIENTED_EDGE('',*,*,#3950,.T.);
#5600=ORIENTED_EDGE('',*,*,#3777,.T.);
#5601=ORIENTED_EDGE('',*,*,#3686,.T.);
#5602=ORIENTED_EDGE('',*,*,#3779,.T.);
#5603=ORIENTED_EDGE('',*,*,#3951,.F.);
#5604=ORIENTED_EDGE('',*,*,#3787,.F.);
#5605=ORIENTED_EDGE('',*,*,#3951,.T.);
#5606=ORIENTED_EDGE('',*,*,#3778,.T.);
#5607=ORIENTED_EDGE('',*,*,#3950,.F.);
#5608=ORIENTED_EDGE('',*,*,#3788,.F.);
#5728=PLANE('',#6700);
#5729=PLANE('',#6705);
#5730=PLANE('',#6708);
#5731=PLANE('',#6710);
#5732=PLANE('',#6714);
#5733=PLANE('',#6718);
#5734=PLANE('',#6722);
#5735=PLANE('',#6726);
#5736=PLANE('',#6730);
#5737=PLANE('',#6734);
#5738=PLANE('',#6738);
#5739=PLANE('',#6744);
#5740=PLANE('',#6745);
#5741=PLANE('',#6753);
#5742=PLANE('',#6757);
#5743=PLANE('',#6761);
#5744=PLANE('',#6765);
#5745=PLANE('',#6769);
#5746=PLANE('',#6773);
#5747=PLANE('',#6777);
#5748=PLANE('',#6781);
#5749=PLANE('',#6801);
#5750=PLANE('',#6804);
#5751=PLANE('',#6807);
#5752=PLANE('',#6810);
#5753=PLANE('',#6813);
#5754=PLANE('',#6816);
#5755=PLANE('',#6819);
#5756=PLANE('',#6822);
#5757=PLANE('',#6825);
#5758=PLANE('',#6826);
#5759=PLANE('',#6827);
#5760=PLANE('',#6828);
#5761=PLANE('',#6830);
#5762=PLANE('',#6831);
#5763=PLANE('',#6832);
#5764=PLANE('',#6833);
#5765=PLANE('',#6835);
#5766=PLANE('',#6836);
#5767=PLANE('',#6837);
#5768=PLANE('',#6838);
#5769=PLANE('',#6840);
#5770=PLANE('',#6841);
#5771=PLANE('',#6842);
#5772=PLANE('',#6843);
#5773=PLANE('',#6844);
#5774=PLANE('',#6845);
#5775=PLANE('',#6846);
#5776=PLANE('',#6847);
#5777=PLANE('',#6848);
#6016=ADVANCED_FACE('',(#967),#566,.F.);
#6017=ADVANCED_FACE('',(#968),#567,.F.);
#6018=ADVANCED_FACE('',(#969),#568,.T.);
#6019=ADVANCED_FACE('',(#970),#569,.T.);
#6020=ADVANCED_FACE('',(#971),#570,.T.);
#6021=ADVANCED_FACE('',(#972),#571,.T.);
#6022=ADVANCED_FACE('',(#973),#572,.T.);
#6023=ADVANCED_FACE('',(#974),#573,.T.);
#6024=ADVANCED_FACE('',(#975),#574,.T.);
#6025=ADVANCED_FACE('',(#976),#575,.T.);
#6026=ADVANCED_FACE('',(#977),#576,.T.);
#6027=ADVANCED_FACE('',(#978),#577,.T.);
#6028=ADVANCED_FACE('',(#979),#578,.T.);
#6029=ADVANCED_FACE('',(#980),#579,.T.);
#6030=ADVANCED_FACE('',(#981),#580,.T.);
#6031=ADVANCED_FACE('',(#982),#581,.T.);
#6032=ADVANCED_FACE('',(#983),#582,.T.);
#6033=ADVANCED_FACE('',(#984),#583,.F.);
#6034=ADVANCED_FACE('',(#985,#687),#5728,.T.);
#6035=ADVANCED_FACE('',(#986,#688),#5729,.F.);
#6036=ADVANCED_FACE('',(#987),#584,.T.);
#6037=ADVANCED_FACE('',(#988,#689),#5730,.F.);
#6038=ADVANCED_FACE('',(#989),#5731,.T.);
#6039=ADVANCED_FACE('',(#990,#690),#5732,.F.);
#6040=ADVANCED_FACE('',(#991),#585,.T.);
#6041=ADVANCED_FACE('',(#992,#691),#5733,.F.);
#6042=ADVANCED_FACE('',(#993),#586,.T.);
#6043=ADVANCED_FACE('',(#994,#692),#5734,.F.);
#6044=ADVANCED_FACE('',(#995),#587,.T.);
#6045=ADVANCED_FACE('',(#996,#693),#5735,.F.);
#6046=ADVANCED_FACE('',(#997),#588,.T.);
#6047=ADVANCED_FACE('',(#998,#694),#5736,.T.);
#6048=ADVANCED_FACE('',(#999),#589,.F.);
#6049=ADVANCED_FACE('',(#1000,#695),#5737,.T.);
#6050=ADVANCED_FACE('',(#1001),#590,.F.);
#6051=ADVANCED_FACE('',(#1002,#696),#5738,.T.);
#6052=ADVANCED_FACE('',(#1003),#591,.F.);
#6053=ADVANCED_FACE('',(#1004,#697,#698,#699,#700,#701,#702,#703,#704,#705,
#706,#707,#708),#592,.F.);
#6054=ADVANCED_FACE('',(#1005),#5739,.F.);
#6055=ADVANCED_FACE('',(#1006,#709),#5740,.T.);
#6056=ADVANCED_FACE('',(#1007),#593,.F.);
#6057=ADVANCED_FACE('',(#1008),#594,.F.);
#6058=ADVANCED_FACE('',(#1009),#595,.F.);
#6059=ADVANCED_FACE('',(#1010),#596,.F.);
#6060=ADVANCED_FACE('',(#1011),#597,.F.);
#6061=ADVANCED_FACE('',(#1012,#710),#5741,.F.);
#6062=ADVANCED_FACE('',(#1013),#598,.T.);
#6063=ADVANCED_FACE('',(#1014,#711),#5742,.F.);
#6064=ADVANCED_FACE('',(#1015),#599,.T.);
#6065=ADVANCED_FACE('',(#1016,#712),#5743,.F.);
#6066=ADVANCED_FACE('',(#1017),#600,.T.);
#6067=ADVANCED_FACE('',(#1018,#713),#5744,.F.);
#6068=ADVANCED_FACE('',(#1019),#601,.T.);
#6069=ADVANCED_FACE('',(#1020,#714),#5745,.F.);
#6070=ADVANCED_FACE('',(#1021),#602,.T.);
#6071=ADVANCED_FACE('',(#1022,#715),#5746,.F.);
#6072=ADVANCED_FACE('',(#1023),#603,.T.);
#6073=ADVANCED_FACE('',(#1024,#716),#5747,.F.);
#6074=ADVANCED_FACE('',(#1025),#604,.T.);
#6075=ADVANCED_FACE('',(#1026,#717),#5748,.F.);
#6076=ADVANCED_FACE('',(#1027),#605,.T.);
#6077=ADVANCED_FACE('',(#1028),#606,.F.);
#6078=ADVANCED_FACE('',(#1029),#607,.F.);
#6079=ADVANCED_FACE('',(#1030),#608,.F.);
#6080=ADVANCED_FACE('',(#1031),#609,.F.);
#6081=ADVANCED_FACE('',(#1032),#610,.F.);
#6082=ADVANCED_FACE('',(#1033),#611,.F.);
#6083=ADVANCED_FACE('',(#1034),#612,.F.);
#6084=ADVANCED_FACE('',(#1035),#613,.F.);
#6085=ADVANCED_FACE('',(#1036,#718),#5749,.T.);
#6086=ADVANCED_FACE('',(#1037),#614,.F.);
#6087=ADVANCED_FACE('',(#1038,#719),#5750,.T.);
#6088=ADVANCED_FACE('',(#1039),#615,.F.);
#6089=ADVANCED_FACE('',(#1040,#720),#5751,.T.);
#6090=ADVANCED_FACE('',(#1041),#616,.F.);
#6091=ADVANCED_FACE('',(#1042,#721),#5752,.T.);
#6092=ADVANCED_FACE('',(#1043),#617,.F.);
#6093=ADVANCED_FACE('',(#1044,#722),#5753,.T.);
#6094=ADVANCED_FACE('',(#1045),#618,.F.);
#6095=ADVANCED_FACE('',(#1046,#723),#5754,.T.);
#6096=ADVANCED_FACE('',(#1047),#619,.F.);
#6097=ADVANCED_FACE('',(#1048,#724),#5755,.T.);
#6098=ADVANCED_FACE('',(#1049),#620,.F.);
#6099=ADVANCED_FACE('',(#1050,#725),#5756,.T.);
#6100=ADVANCED_FACE('',(#1051),#621,.F.);
#6101=ADVANCED_FACE('',(#1052),#5757,.F.);
#6102=ADVANCED_FACE('',(#1053),#5758,.F.);
#6103=ADVANCED_FACE('',(#1054),#5759,.T.);
#6104=ADVANCED_FACE('',(#1055),#5760,.T.);
#6105=ADVANCED_FACE('',(#1056),#289,.T.);
#6106=ADVANCED_FACE('',(#1057,#726),#622,.T.);
#6107=ADVANCED_FACE('',(#1058),#5761,.F.);
#6108=ADVANCED_FACE('',(#1059),#5762,.F.);
#6109=ADVANCED_FACE('',(#1060),#5763,.T.);
#6110=ADVANCED_FACE('',(#1061),#5764,.T.);
#6111=ADVANCED_FACE('',(#1062),#290,.T.);
#6112=ADVANCED_FACE('',(#1063,#727),#623,.T.);
#6113=ADVANCED_FACE('',(#1064),#5765,.F.);
#6114=ADVANCED_FACE('',(#1065),#5766,.F.);
#6115=ADVANCED_FACE('',(#1066),#5767,.T.);
#6116=ADVANCED_FACE('',(#1067),#5768,.T.);
#6117=ADVANCED_FACE('',(#1068),#291,.T.);
#6118=ADVANCED_FACE('',(#1069,#728),#624,.T.);
#6119=ADVANCED_FACE('',(#1070),#5769,.F.);
#6120=ADVANCED_FACE('',(#1071),#5770,.F.);
#6121=ADVANCED_FACE('',(#1072),#5771,.F.);
#6122=ADVANCED_FACE('',(#1073),#5772,.F.);
#6123=ADVANCED_FACE('',(#1074),#5773,.F.);
#6124=ADVANCED_FACE('',(#1075),#5774,.F.);
#6125=ADVANCED_FACE('',(#1076),#5775,.F.);
#6126=ADVANCED_FACE('',(#1077),#5776,.F.);
#6127=ADVANCED_FACE('',(#1078),#5777,.F.);
#6145=CLOSED_SHELL('',(#6016,#6017,#6018,#6019,#6020,#6021,#6022,#6023,
#6024,#6025,#6026,#6027,#6028,#6029,#6030,#6031,#6032,#6033,#6034,#6035,
#6036,#6037,#6038,#6039,#6040,#6041,#6042,#6043,#6044,#6045,#6046,#6047,
#6048,#6049,#6050,#6051,#6052,#6053,#6054,#6055,#6056,#6057,#6058,#6059,
#6060,#6061,#6062,#6063,#6064,#6065,#6066,#6067,#6068,#6069,#6070,#6071,
#6072,#6073,#6074,#6075,#6076,#6077,#6078,#6079,#6080,#6081,#6082,#6083,
#6084,#6085,#6086,#6087,#6088,#6089,#6090,#6091,#6092,#6093,#6094,#6095,
#6096,#6097,#6098,#6099,#6100,#6101,#6102,#6103,#6104,#6105,#6106,#6107,
#6108,#6109,#6110,#6111,#6112,#6113,#6114,#6115,#6116,#6117,#6118,#6119,
#6120,#6121,#6122,#6123,#6124,#6125,#6126,#6127));
#6669=AXIS2_PLACEMENT_3D('',#12317,#7980,#7981);
#6670=AXIS2_PLACEMENT_3D('',#12318,#7982,#7983);
#6671=AXIS2_PLACEMENT_3D('',#12323,#7985,#7986);
#6672=AXIS2_PLACEMENT_3D('',#12326,#7988,#7989);
#6673=AXIS2_PLACEMENT_3D('',#12327,#7990,#7991);
#6674=AXIS2_PLACEMENT_3D('',#12332,#7993,#7994);
#6675=AXIS2_PLACEMENT_3D('',#12335,#7996,#7997);
#6676=AXIS2_PLACEMENT_3D('',#12336,#7998,#7999);
#6677=AXIS2_PLACEMENT_3D('',#12339,#8000,#8001);
#6678=AXIS2_PLACEMENT_3D('',#12343,#8003,#8004);
#6679=AXIS2_PLACEMENT_3D('',#12345,#8006,#8007);
#6680=AXIS2_PLACEMENT_3D('',#12398,#8010,#8011);
#6681=AXIS2_PLACEMENT_3D('',#12444,#8014,#8015);
#6682=AXIS2_PLACEMENT_3D('',#12490,#8018,#8019);
#6683=AXIS2_PLACEMENT_3D('',#12543,#8022,#8023);
#6684=AXIS2_PLACEMENT_3D('',#12546,#8024,#8025);
#6685=AXIS2_PLACEMENT_3D('',#12550,#8027,#8028);
#6686=AXIS2_PLACEMENT_3D('',#12552,#8030,#8031);
#6687=AXIS2_PLACEMENT_3D('',#12605,#8034,#8035);
#6688=AXIS2_PLACEMENT_3D('',#12651,#8038,#8039);
#6689=AXIS2_PLACEMENT_3D('',#12697,#8042,#8043);
#6690=AXIS2_PLACEMENT_3D('',#12750,#8046,#8047);
#6691=AXIS2_PLACEMENT_3D('',#12803,#8050,#8051);
#6692=AXIS2_PLACEMENT_3D('',#12849,#8054,#8055);
#6693=AXIS2_PLACEMENT_3D('',#12895,#8058,#8059);
#6694=AXIS2_PLACEMENT_3D('',#12948,#8062,#8063);
#6695=AXIS2_PLACEMENT_3D('',#12951,#8064,#8065);
#6696=AXIS2_PLACEMENT_3D('',#12955,#8067,#8068);
#6697=AXIS2_PLACEMENT_3D('',#12957,#8070,#8071);
#6698=AXIS2_PLACEMENT_3D('',#12962,#8073,#8074);
#6699=AXIS2_PLACEMENT_3D('',#12965,#8076,#8077);
#6700=AXIS2_PLACEMENT_3D('',#12966,#8078,#8079);
#6701=AXIS2_PLACEMENT_3D('',#12968,#8080,#8081);
#6702=AXIS2_PLACEMENT_3D('',#12972,#8083,#8084);
#6703=AXIS2_PLACEMENT_3D('',#12977,#8087,#8088);
#6704=AXIS2_PLACEMENT_3D('',#12982,#8091,#8092);
#6705=AXIS2_PLACEMENT_3D('',#12984,#8094,#8095);
#6706=AXIS2_PLACEMENT_3D('',#12986,#8096,#8097);
#6707=AXIS2_PLACEMENT_3D('',#13002,#8107,#8108);
#6708=AXIS2_PLACEMENT_3D('',#13004,#8110,#8111);
#6709=AXIS2_PLACEMENT_3D('',#13021,#8121,#8122);
#6710=AXIS2_PLACEMENT_3D('',#13022,#8123,#8124);
#6711=AXIS2_PLACEMENT_3D('',#13026,#8126,#8127);
#6712=AXIS2_PLACEMENT_3D('',#13031,#8130,#8131);
#6713=AXIS2_PLACEMENT_3D('',#13036,#8134,#8135);
#6714=AXIS2_PLACEMENT_3D('',#13038,#8137,#8138);
#6715=AXIS2_PLACEMENT_3D('',#13040,#8139,#8140);
#6716=AXIS2_PLACEMENT_3D('',#13042,#8141,#8142);
#6717=AXIS2_PLACEMENT_3D('',#13043,#8143,#8144);
#6718=AXIS2_PLACEMENT_3D('',#13067,#8148,#8149);
#6719=AXIS2_PLACEMENT_3D('',#13069,#8150,#8151);
#6720=AXIS2_PLACEMENT_3D('',#13071,#8152,#8153);
#6721=AXIS2_PLACEMENT_3D('',#13072,#8154,#8155);
#6722=AXIS2_PLACEMENT_3D('',#13074,#8157,#8158);
#6723=AXIS2_PLACEMENT_3D('',#13076,#8159,#8160);
#6724=AXIS2_PLACEMENT_3D('',#13078,#8161,#8162);
#6725=AXIS2_PLACEMENT_3D('',#13079,#8163,#8164);
#6726=AXIS2_PLACEMENT_3D('',#13081,#8166,#8167);
#6727=AXIS2_PLACEMENT_3D('',#13083,#8168,#8169);
#6728=AXIS2_PLACEMENT_3D('',#13085,#8170,#8171);
#6729=AXIS2_PLACEMENT_3D('',#13086,#8172,#8173);
#6730=AXIS2_PLACEMENT_3D('',#13088,#8175,#8176);
#6731=AXIS2_PLACEMENT_3D('',#13090,#8177,#8178);
#6732=AXIS2_PLACEMENT_3D('',#13092,#8179,#8180);
#6733=AXIS2_PLACEMENT_3D('',#13093,#8181,#8182);
#6734=AXIS2_PLACEMENT_3D('',#13095,#8184,#8185);
#6735=AXIS2_PLACEMENT_3D('',#13097,#8186,#8187);
#6736=AXIS2_PLACEMENT_3D('',#13099,#8188,#8189);
#6737=AXIS2_PLACEMENT_3D('',#13100,#8190,#8191);
#6738=AXIS2_PLACEMENT_3D('',#13102,#8193,#8194);
#6739=AXIS2_PLACEMENT_3D('',#13104,#8195,#8196);
#6740=AXIS2_PLACEMENT_3D('',#13106,#8197,#8198);
#6741=AXIS2_PLACEMENT_3D('',#13107,#8199,#8200);
#6742=AXIS2_PLACEMENT_3D('',#13109,#8202,#8203);
#6743=AXIS2_PLACEMENT_3D('',#13111,#8204,#8205);
#6744=AXIS2_PLACEMENT_3D('',#13641,#8207,#8208);
#6745=AXIS2_PLACEMENT_3D('',#13642,#8209,#8210);
#6746=AXIS2_PLACEMENT_3D('',#13644,#8211,#8212);
#6747=AXIS2_PLACEMENT_3D('',#13646,#8213,#8214);
#6748=AXIS2_PLACEMENT_3D('',#13647,#8215,#8216);
#6749=AXIS2_PLACEMENT_3D('',#13649,#8218,#8219);
#6750=AXIS2_PLACEMENT_3D('',#13651,#8221,#8222);
#6751=AXIS2_PLACEMENT_3D('',#13653,#8224,#8225);
#6752=AXIS2_PLACEMENT_3D('',#13655,#8227,#8228);
#6753=AXIS2_PLACEMENT_3D('',#13657,#8230,#8231);
#6754=AXIS2_PLACEMENT_3D('',#13659,#8232,#8233);
#6755=AXIS2_PLACEMENT_3D('',#13661,#8234,#8235);
#6756=AXIS2_PLACEMENT_3D('',#13662,#8236,#8237);
#6757=AXIS2_PLACEMENT_3D('',#13686,#8241,#8242);
#6758=AXIS2_PLACEMENT_3D('',#13688,#8243,#8244);
#6759=AXIS2_PLACEMENT_3D('',#13690,#8245,#8246);
#6760=AXIS2_PLACEMENT_3D('',#13691,#8247,#8248);
#6761=AXIS2_PLACEMENT_3D('',#13715,#8252,#8253);
#6762=AXIS2_PLACEMENT_3D('',#13717,#8254,#8255);
#6763=AXIS2_PLACEMENT_3D('',#13719,#8256,#8257);
#6764=AXIS2_PLACEMENT_3D('',#13720,#8258,#8259);
#6765=AXIS2_PLACEMENT_3D('',#13722,#8261,#8262);
#6766=AXIS2_PLACEMENT_3D('',#13724,#8263,#8264);
#6767=AXIS2_PLACEMENT_3D('',#13726,#8265,#8266);
#6768=AXIS2_PLACEMENT_3D('',#13727,#8267,#8268);
#6769=AXIS2_PLACEMENT_3D('',#13729,#8270,#8271);
#6770=AXIS2_PLACEMENT_3D('',#13731,#8272,#8273);
#6771=AXIS2_PLACEMENT_3D('',#13733,#8274,#8275);
#6772=AXIS2_PLACEMENT_3D('',#13734,#8276,#8277);
#6773=AXIS2_PLACEMENT_3D('',#13736,#8279,#8280);
#6774=AXIS2_PLACEMENT_3D('',#13738,#8281,#8282);
#6775=AXIS2_PLACEMENT_3D('',#13740,#8283,#8284);
#6776=AXIS2_PLACEMENT_3D('',#13741,#8285,#8286);
#6777=AXIS2_PLACEMENT_3D('',#13743,#8288,#8289);
#6778=AXIS2_PLACEMENT_3D('',#13745,#8290,#8291);
#6779=AXIS2_PLACEMENT_3D('',#13747,#8292,#8293);
#6780=AXIS2_PLACEMENT_3D('',#13748,#8294,#8295);
#6781=AXIS2_PLACEMENT_3D('',#13750,#8297,#8298);
#6782=AXIS2_PLACEMENT_3D('',#13752,#8299,#8300);
#6783=AXIS2_PLACEMENT_3D('',#13754,#8301,#8302);
#6784=AXIS2_PLACEMENT_3D('',#13755,#8303,#8304);
#6785=AXIS2_PLACEMENT_3D('',#13757,#8306,#8307);
#6786=AXIS2_PLACEMENT_3D('',#13760,#8309,#8310);
#6787=AXIS2_PLACEMENT_3D('',#13761,#8311,#8312);
#6788=AXIS2_PLACEMENT_3D('',#13764,#8314,#8315);
#6789=AXIS2_PLACEMENT_3D('',#13765,#8316,#8317);
#6790=AXIS2_PLACEMENT_3D('',#13768,#8319,#8320);
#6791=AXIS2_PLACEMENT_3D('',#13769,#8321,#8322);
#6792=AXIS2_PLACEMENT_3D('',#13772,#8324,#8325);
#6793=AXIS2_PLACEMENT_3D('',#13773,#8326,#8327);
#6794=AXIS2_PLACEMENT_3D('',#13776,#8329,#8330);
#6795=AXIS2_PLACEMENT_3D('',#13777,#8331,#8332);
#6796=AXIS2_PLACEMENT_3D('',#13780,#8334,#8335);
#6797=AXIS2_PLACEMENT_3D('',#13781,#8336,#8337);
#6798=AXIS2_PLACEMENT_3D('',#13784,#8339,#8340);
#6799=AXIS2_PLACEMENT_3D('',#13785,#8341,#8342);
#6800=AXIS2_PLACEMENT_3D('',#13788,#8344,#8345);
#6801=AXIS2_PLACEMENT_3D('',#13789,#8346,#8347);
#6802=AXIS2_PLACEMENT_3D('',#13791,#8348,#8349);
#6803=AXIS2_PLACEMENT_3D('',#13792,#8350,#8351);
#6804=AXIS2_PLACEMENT_3D('',#13794,#8353,#8354);
#6805=AXIS2_PLACEMENT_3D('',#13796,#8355,#8356);
#6806=AXIS2_PLACEMENT_3D('',#13797,#8357,#8358);
#6807=AXIS2_PLACEMENT_3D('',#13799,#8360,#8361);
#6808=AXIS2_PLACEMENT_3D('',#13801,#8362,#8363);
#6809=AXIS2_PLACEMENT_3D('',#13802,#8364,#8365);
#6810=AXIS2_PLACEMENT_3D('',#13804,#8367,#8368);
#6811=AXIS2_PLACEMENT_3D('',#13806,#8369,#8370);
#6812=AXIS2_PLACEMENT_3D('',#13807,#8371,#8372);
#6813=AXIS2_PLACEMENT_3D('',#13809,#8374,#8375);
#6814=AXIS2_PLACEMENT_3D('',#13811,#8376,#8377);
#6815=AXIS2_PLACEMENT_3D('',#13812,#8378,#8379);
#6816=AXIS2_PLACEMENT_3D('',#13814,#8381,#8382);
#6817=AXIS2_PLACEMENT_3D('',#13816,#8383,#8384);
#6818=AXIS2_PLACEMENT_3D('',#13817,#8385,#8386);
#6819=AXIS2_PLACEMENT_3D('',#13819,#8388,#8389);
#6820=AXIS2_PLACEMENT_3D('',#13821,#8390,#8391);
#6821=AXIS2_PLACEMENT_3D('',#13822,#8392,#8393);
#6822=AXIS2_PLACEMENT_3D('',#13824,#8395,#8396);
#6823=AXIS2_PLACEMENT_3D('',#13826,#8397,#8398);
#6824=AXIS2_PLACEMENT_3D('',#13827,#8399,#8400);
#6825=AXIS2_PLACEMENT_3D('',#13829,#8402,#8403);
#6826=AXIS2_PLACEMENT_3D('',#13831,#8405,#8406);
#6827=AXIS2_PLACEMENT_3D('',#13833,#8408,#8409);
#6828=AXIS2_PLACEMENT_3D('',#13837,#8412,#8413);
#6829=AXIS2_PLACEMENT_3D('',#13891,#8416,#8417);
#6830=AXIS2_PLACEMENT_3D('',#13892,#8418,#8419);
#6831=AXIS2_PLACEMENT_3D('',#13894,#8421,#8422);
#6832=AXIS2_PLACEMENT_3D('',#13896,#8424,#8425);
#6833=AXIS2_PLACEMENT_3D('',#13900,#8428,#8429);
#6834=AXIS2_PLACEMENT_3D('',#13954,#8432,#8433);
#6835=AXIS2_PLACEMENT_3D('',#13955,#8434,#8435);
#6836=AXIS2_PLACEMENT_3D('',#13957,#8437,#8438);
#6837=AXIS2_PLACEMENT_3D('',#13959,#8440,#8441);
#6838=AXIS2_PLACEMENT_3D('',#13963,#8444,#8445);
#6839=AXIS2_PLACEMENT_3D('',#14017,#8448,#8449);
#6840=AXIS2_PLACEMENT_3D('',#14018,#8450,#8451);
#6841=AXIS2_PLACEMENT_3D('',#14020,#8453,#8454);
#6842=AXIS2_PLACEMENT_3D('',#14022,#8456,#8457);
#6843=AXIS2_PLACEMENT_3D('',#14023,#8458,#8459);
#6844=AXIS2_PLACEMENT_3D('',#14025,#8461,#8462);
#6845=AXIS2_PLACEMENT_3D('',#14027,#8464,#8465);
#6846=AXIS2_PLACEMENT_3D('',#14028,#8466,#8467);
#6847=AXIS2_PLACEMENT_3D('',#14030,#8469,#8470);
#6848=AXIS2_PLACEMENT_3D('',#14032,#8472,#8473);
#7980=DIRECTION('axis',(0.,0.,1.));
#7981=DIRECTION('refdir',(1.,0.,0.));
#7982=DIRECTION('center_axis',(0.866025403784443,0.,0.499999999999992));
#7983=DIRECTION('ref_axis',(0.499999999999992,0.,-0.866025403784443));
#7984=DIRECTION('',(0.866025403784444,0.,0.499999999999991));
#7985=DIRECTION('center_axis',(-0.866025403784443,0.,-0.499999999999992));
#7986=DIRECTION('ref_axis',(-0.499999999999992,0.,0.866025403784443));
#7987=DIRECTION('',(0.866025403784443,0.,0.499999999999992));
#7988=DIRECTION('center_axis',(-0.866025403784443,0.,-0.499999999999992));
#7989=DIRECTION('ref_axis',(-0.499999999999992,0.,0.866025403784443));
#7990=DIRECTION('center_axis',(0.866025403784443,0.,0.499999999999992));
#7991=DIRECTION('ref_axis',(0.499999999999992,0.,-0.866025403784443));
#7992=DIRECTION('',(0.866025403784443,0.,0.499999999999993));
#7993=DIRECTION('center_axis',(-0.866025403784443,0.,-0.499999999999992));
#7994=DIRECTION('ref_axis',(-0.499999999999992,0.,0.866025403784443));
#7995=DIRECTION('',(0.866025403784443,0.,0.499999999999993));
#7996=DIRECTION('center_axis',(-0.866025403784443,0.,-0.499999999999992));
#7997=DIRECTION('ref_axis',(-0.499999999999992,0.,0.866025403784443));
#7998=DIRECTION('center_axis',(0.866025403784443,0.,0.499999999999992));
#7999=DIRECTION('ref_axis',(0.499999999999992,0.,-0.866025403784443));
#8000=DIRECTION('center_axis',(-0.866025403784443,0.,-0.499999999999992));
#8001=DIRECTION('ref_axis',(-0.499999999999992,0.,0.866025403784443));
#8002=DIRECTION('',(0.866025403784443,0.,0.499999999999992));
#8003=DIRECTION('center_axis',(-0.866025403784443,0.,-0.499999999999992));
#8004=DIRECTION('ref_axis',(-0.499999999999992,0.,0.866025403784443));
#8005=DIRECTION('',(0.866025403784443,0.,0.499999999999992));
#8006=DIRECTION('center_axis',(0.866025403784443,0.,0.499999999999992));
#8007=DIRECTION('ref_axis',(0.499999999999992,0.,-0.866025403784443));
#8008=DIRECTION('',(0.866025403784443,0.,0.499999999999992));
#8009=DIRECTION('',(0.866025403784443,0.,0.499999999999992));
#8010=DIRECTION('center_axis',(0.866025403784443,0.,0.499999999999992));
#8011=DIRECTION('ref_axis',(0.499999999999992,0.,-0.866025403784443));
#8012=DIRECTION('',(0.866025403784443,0.,0.499999999999992));
#8013=DIRECTION('',(0.866025403784443,0.,0.499999999999992));
#8014=DIRECTION('center_axis',(0.866025403784443,0.,0.499999999999992));
#8015=DIRECTION('ref_axis',(0.499999999999992,0.,-0.866025403784443));
#8016=DIRECTION('',(0.866025403784444,0.,0.499999999999991));
#8017=DIRECTION('',(0.866025403784443,0.,0.499999999999992));
#8018=DIRECTION('center_axis',(0.866025403784443,0.,0.499999999999992));
#8019=DIRECTION('ref_axis',(0.499999999999992,0.,-0.866025403784443));
#8020=DIRECTION('',(0.866025403784443,0.,0.499999999999993));
#8021=DIRECTION('',(0.866025403784443,0.,0.499999999999992));
#8022=DIRECTION('center_axis',(0.866025403784443,0.,0.499999999999992));
#8023=DIRECTION('ref_axis',(0.499999999999992,0.,-0.866025403784443));
#8024=DIRECTION('center_axis',(-0.866025403784443,0.,-0.499999999999992));
#8025=DIRECTION('ref_axis',(-0.499999999999992,0.,0.866025403784443));
#8026=DIRECTION('',(0.866025403784443,0.,0.499999999999992));
#8027=DIRECTION('center_axis',(-0.866025403784443,0.,-0.499999999999992));
#8028=DIRECTION('ref_axis',(-0.499999999999992,0.,0.866025403784443));
#8029=DIRECTION('',(0.866025403784443,0.,0.499999999999992));
#8030=DIRECTION('center_axis',(0.866025403784443,0.,0.499999999999992));
#8031=DIRECTION('ref_axis',(0.499999999999992,0.,-0.866025403784443));
#8032=DIRECTION('',(0.866025403784443,0.,0.499999999999992));
#8033=DIRECTION('',(0.866025403784443,0.,0.499999999999993));
#8034=DIRECTION('center_axis',(0.866025403784443,0.,0.499999999999992));
#8035=DIRECTION('ref_axis',(0.499999999999992,0.,-0.866025403784443));
#8036=DIRECTION('',(0.866025403784444,0.,0.499999999999991));
#8037=DIRECTION('',(0.866025403784443,0.,0.499999999999992));
#8038=DIRECTION('center_axis',(0.866025403784443,0.,0.499999999999992));
#8039=DIRECTION('ref_axis',(0.499999999999992,0.,-0.866025403784443));
#8040=DIRECTION('',(0.866025403784443,0.,0.499999999999992));
#8041=DIRECTION('',(0.866025403784443,0.,0.499999999999992));
#8042=DIRECTION('center_axis',(0.866025403784443,0.,0.499999999999992));
#8043=DIRECTION('ref_axis',(0.499999999999992,0.,-0.866025403784443));
#8044=DIRECTION('',(0.866025403784444,0.,0.49999999999999));
#8045=DIRECTION('',(0.866025403784441,0.,0.499999999999995));
#8046=DIRECTION('center_axis',(0.866025403784443,0.,0.499999999999992));
#8047=DIRECTION('ref_axis',(0.499999999999992,0.,-0.866025403784443));
#8048=DIRECTION('',(0.866025403784443,0.,0.499999999999993));
#8049=DIRECTION('',(0.866025403784443,0.,0.499999999999992));
#8050=DIRECTION('center_axis',(0.866025403784443,0.,0.499999999999992));
#8051=DIRECTION('ref_axis',(0.499999999999992,0.,-0.866025403784443));
#8052=DIRECTION('',(0.866025403784443,0.,0.499999999999992));
#8053=DIRECTION('',(0.866025403784443,0.,0.499999999999992));
#8054=DIRECTION('center_axis',(0.866025403784443,0.,0.499999999999992));
#8055=DIRECTION('ref_axis',(0.499999999999992,0.,-0.866025403784443));
#8056=DIRECTION('',(0.866025403784443,0.,0.499999999999992));
#8057=DIRECTION('',(0.866025403784443,0.,0.499999999999992));
#8058=DIRECTION('center_axis',(0.866025403784443,0.,0.499999999999992));
#8059=DIRECTION('ref_axis',(0.499999999999992,0.,-0.866025403784443));
#8060=DIRECTION('',(0.866025403784443,0.,0.499999999999992));
#8061=DIRECTION('',(0.866025403784444,0.,0.499999999999991));
#8062=DIRECTION('center_axis',(0.866025403784443,0.,0.499999999999992));
#8063=DIRECTION('ref_axis',(-0.433012701892211,0.500000000000004,0.750000000000002));
#8064=DIRECTION('center_axis',(-0.866025403784443,0.,-0.499999999999992));
#8065=DIRECTION('ref_axis',(-0.499999999999992,0.,0.866025403784443));
#8066=DIRECTION('',(0.866025403784443,0.,0.499999999999992));
#8067=DIRECTION('center_axis',(-0.866025403784443,0.,-0.499999999999992));
#8068=DIRECTION('ref_axis',(-0.499999999999992,0.,0.866025403784443));
#8069=DIRECTION('',(0.866025403784443,0.,0.499999999999992));
#8070=DIRECTION('center_axis',(0.866025403784443,0.,0.499999999999992));
#8071=DIRECTION('ref_axis',(-0.433012701892234,0.499999999999926,0.750000000000041));
#8072=DIRECTION('',(0.866025403784443,0.,0.499999999999992));
#8073=DIRECTION('center_axis',(-0.866025403784443,0.,-0.499999999999992));
#8074=DIRECTION('ref_axis',(-0.499999999999992,0.,0.866025403784443));
#8075=DIRECTION('',(0.866025403784442,0.,0.499999999999994));
#8076=DIRECTION('center_axis',(-0.866025403784443,0.,-0.499999999999992));
#8077=DIRECTION('ref_axis',(-0.499999999999992,0.,0.866025403784443));
#8078=DIRECTION('center_axis',(-0.866025403784443,0.,-0.499999999999992));
#8079=DIRECTION('ref_axis',(-0.499999999999992,0.,0.866025403784443));
#8080=DIRECTION('center_axis',(-0.866025403784443,0.,-0.499999999999992));
#8081=DIRECTION('ref_axis',(-0.499999999999992,0.,0.866025403784443));
#8082=DIRECTION('',(-0.433012701892229,-0.499999999999983,0.750000000000006));
#8083=DIRECTION('center_axis',(0.866025403784443,-2.25118642417821E-16,
0.499999999999992));
#8084=DIRECTION('ref_axis',(0.499999999999992,0.,-0.866025403784443));
#8085=DIRECTION('',(-0.433012701892221,-0.499999999999992,0.750000000000004));
#8086=DIRECTION('',(0.433012701892197,-0.500000000000028,-0.749999999999994));
#8087=DIRECTION('center_axis',(0.866025403784443,2.4704687096211E-16,0.499999999999992));
#8088=DIRECTION('ref_axis',(0.499999999999992,0.,-0.866025403784443));
#8089=DIRECTION('',(0.433012701892204,-0.500000000000004,-0.750000000000006));
#8090=DIRECTION('',(0.,1.,0.));
#8091=DIRECTION('center_axis',(0.866025403784443,0.,0.499999999999992));
#8092=DIRECTION('ref_axis',(0.499999999999992,0.,-0.866025403784443));
#8093=DIRECTION('',(0.,1.,0.));
#8094=DIRECTION('center_axis',(-0.866025403784443,0.,-0.499999999999992));
#8095=DIRECTION('ref_axis',(-0.499999999999992,0.,0.866025403784443));
#8096=DIRECTION('center_axis',(-0.866025403784443,0.,-0.499999999999992));
#8097=DIRECTION('ref_axis',(-0.499999999999992,0.,0.866025403784443));
#8098=DIRECTION('',(-0.43301270189221,0.500000000000002,0.750000000000004));
#8099=DIRECTION('',(0.25,0.866025403784439,-0.433012701892219));
#8100=DIRECTION('',(0.433012701892205,-0.500000000000012,-0.75));
#8101=DIRECTION('',(0.433012701892215,0.499999999999987,-0.750000000000011));
#8102=DIRECTION('',(0.25,-0.86602540378444,-0.433012701892216));
#8103=DIRECTION('',(-0.433012701892207,-0.499999999999993,0.750000000000012));
#8104=DIRECTION('',(0.,-1.,0.));
#8105=DIRECTION('',(-0.499999999999994,0.,0.866025403784442));
#8106=DIRECTION('',(0.,1.,0.));
#8107=DIRECTION('center_axis',(0.866025403784443,0.,0.499999999999992));
#8108=DIRECTION('ref_axis',(0.499999999999992,0.,-0.866025403784443));
#8109=DIRECTION('',(-0.866025403784443,0.,-0.499999999999992));
#8110=DIRECTION('center_axis',(-0.866025403784443,0.,-0.499999999999992));
#8111=DIRECTION('ref_axis',(-0.499999999999992,0.,0.866025403784443));
#8112=DIRECTION('',(0.433012701892209,-0.500000000000007,-0.750000000000001));
#8113=DIRECTION('',(0.250000000000001,0.866025403784442,-0.433012701892212));
#8114=DIRECTION('',(-0.433012701892215,0.499999999999997,0.750000000000005));
#8115=DIRECTION('',(0.,1.,0.));
#8116=DIRECTION('',(-0.499999999999994,0.,0.866025403784442));
#8117=DIRECTION('',(0.,-1.,0.));
#8118=DIRECTION('',(-0.433012701892214,-0.499999999999991,0.750000000000009));
#8119=DIRECTION('',(0.249999999999992,-0.866025403784442,-0.433012701892217));
#8120=DIRECTION('',(0.433012701892219,0.499999999999982,-0.750000000000012));
#8121=DIRECTION('center_axis',(0.866025403784443,0.,0.499999999999992));
#8122=DIRECTION('ref_axis',(0.499999999999992,0.,-0.866025403784443));
#8123=DIRECTION('center_axis',(-0.866025403784443,0.,-0.499999999999992));
#8124=DIRECTION('ref_axis',(-0.499999999999992,0.,0.866025403784443));
#8125=DIRECTION('',(-0.433012701892211,-0.49999999999998,0.750000000000018));
#8126=DIRECTION('center_axis',(-0.866025403784443,0.,-0.499999999999992));
#8127=DIRECTION('ref_axis',(-0.499999999999992,0.,0.866025403784443));
#8128=DIRECTION('',(0.433012701892242,0.49999999999998,-0.750000000000001));
#8129=DIRECTION('',(0.,1.,0.));
#8130=DIRECTION('center_axis',(-0.866025403784443,0.,-0.499999999999992));
#8131=DIRECTION('ref_axis',(-0.499999999999992,0.,0.866025403784443));
#8132=DIRECTION('',(0.,-1.,0.));
#8133=DIRECTION('',(0.433012701892204,-0.500000000000004,-0.750000000000006));
#8134=DIRECTION('center_axis',(-0.866025403784443,0.,-0.499999999999992));
#8135=DIRECTION('ref_axis',(-0.499999999999992,0.,0.866025403784443));
#8136=DIRECTION('',(-0.433012701892195,0.499999999999999,0.750000000000015));
#8137=DIRECTION('center_axis',(0.,-1.,0.));
#8138=DIRECTION('ref_axis',(0.,0.,-1.));
#8139=DIRECTION('center_axis',(0.,-1.,0.));
#8140=DIRECTION('ref_axis',(0.,0.,-1.));
#8141=DIRECTION('center_axis',(0.,1.,0.));
#8142=DIRECTION('ref_axis',(0.,0.,1.));
#8143=DIRECTION('center_axis',(0.,1.,0.));
#8144=DIRECTION('ref_axis',(0.,0.,1.));
#8145=DIRECTION('',(0.,-1.,0.));
#8146=DIRECTION('',(0.,1.,0.));
#8147=DIRECTION('',(0.,1.,0.));
#8148=DIRECTION('center_axis',(0.224143868042018,-0.965925826289067,0.129409522551263));
#8149=DIRECTION('ref_axis',(0.,-0.132788176096111,-0.991144439670156));
#8150=DIRECTION('center_axis',(0.224143868042018,-0.965925826289067,0.129409522551263));
#8151=DIRECTION('ref_axis',(0.974116947696296,0.22604462437946,0.));
#8152=DIRECTION('center_axis',(-0.224143868042018,0.965925826289067,-0.129409522551263));
#8153=DIRECTION('ref_axis',(-0.974116947696296,-0.22604462437946,0.));
#8154=DIRECTION('center_axis',(-0.224143868042018,0.965925826289067,-0.129409522551263));
#8155=DIRECTION('ref_axis',(-0.974116947696296,-0.22604462437946,0.));
#8156=DIRECTION('',(0.224143868042018,-0.965925826289067,0.129409522551263));
#8157=DIRECTION('center_axis',(0.433012701892223,-0.866025403784436,0.250000000000002));
#8158=DIRECTION('ref_axis',(0.5,0.,-0.866025403784439));
#8159=DIRECTION('center_axis',(0.433012701892223,-0.866025403784436,0.250000000000002));
#8160=DIRECTION('ref_axis',(0.894427190999914,0.447213595499962,0.));
#8161=DIRECTION('center_axis',(-0.433012701892223,0.866025403784436,-0.250000000000002));
#8162=DIRECTION('ref_axis',(-0.894427190999914,-0.447213595499962,0.));
#8163=DIRECTION('center_axis',(-0.433012701892223,0.866025403784436,-0.250000000000002));
#8164=DIRECTION('ref_axis',(-0.894427190999914,-0.447213595499962,0.));
#8165=DIRECTION('',(0.433012701892223,-0.866025403784437,0.250000000000002));
#8166=DIRECTION('center_axis',(0.612372435695796,-0.707106781186546,0.353553390593275));
#8167=DIRECTION('ref_axis',(0.5,0.,-0.866025403784438));
#8168=DIRECTION('center_axis',(0.612372435695796,-0.707106781186546,0.353553390593275));
#8169=DIRECTION('ref_axis',(0.755928946018453,0.654653670707979,0.));
#8170=DIRECTION('center_axis',(-0.612372435695796,0.707106781186546,-0.353553390593275));
#8171=DIRECTION('ref_axis',(-0.755928946018453,-0.654653670707979,0.));
#8172=DIRECTION('center_axis',(-0.612372435695796,0.707106781186546,-0.353553390593275));
#8173=DIRECTION('ref_axis',(-0.755928946018453,-0.654653670707979,0.));
#8174=DIRECTION('',(0.612372435695796,-0.707106781186546,0.353553390593275));
#8175=DIRECTION('center_axis',(0.,1.,0.));
#8176=DIRECTION('ref_axis',(0.,0.,1.));
#8177=DIRECTION('center_axis',(0.,1.,0.));
#8178=DIRECTION('ref_axis',(0.,0.,1.));
#8179=DIRECTION('center_axis',(0.,1.,0.));
#8180=DIRECTION('ref_axis',(0.,0.,1.));
#8181=DIRECTION('center_axis',(0.,1.,0.));
#8182=DIRECTION('ref_axis',(0.,0.,1.));
#8183=DIRECTION('',(0.,1.,0.));
#8184=DIRECTION('center_axis',(-0.224143868042018,0.965925826289067,-0.129409522551263));
#8185=DIRECTION('ref_axis',(0.,0.132788176096111,0.991144439670156));
#8186=DIRECTION('center_axis',(-0.224143868042018,0.965925826289067,-0.129409522551263));
#8187=DIRECTION('ref_axis',(-0.974116947696296,-0.22604462437946,0.));
#8188=DIRECTION('center_axis',(-0.224143868042018,0.965925826289067,-0.129409522551263));
#8189=DIRECTION('ref_axis',(-0.974116947696296,-0.22604462437946,0.));
#8190=DIRECTION('center_axis',(-0.224143868042018,0.965925826289067,-0.129409522551263));
#8191=DIRECTION('ref_axis',(-0.974116947696296,-0.22604462437946,0.));
#8192=DIRECTION('',(-0.224143868042018,0.965925826289067,-0.129409522551263));
#8193=DIRECTION('center_axis',(-0.433012701892223,0.866025403784436,-0.250000000000002));
#8194=DIRECTION('ref_axis',(-0.499999999999999,0.,0.866025403784439));
#8195=DIRECTION('center_axis',(-0.433012701892223,0.866025403784436,-0.250000000000002));
#8196=DIRECTION('ref_axis',(-0.894427190999914,-0.447213595499962,0.));
#8197=DIRECTION('center_axis',(-0.433012701892223,0.866025403784436,-0.250000000000002));
#8198=DIRECTION('ref_axis',(-0.894427190999914,-0.447213595499962,0.));
#8199=DIRECTION('center_axis',(-0.433012701892223,0.866025403784436,-0.250000000000002));
#8200=DIRECTION('ref_axis',(-0.894427190999914,-0.447213595499962,0.));
#8201=DIRECTION('',(-0.433012701892223,0.866025403784436,-0.250000000000002));
#8202=DIRECTION('center_axis',(0.866025403784443,0.,0.499999999999992));
#8203=DIRECTION('ref_axis',(0.499999999999992,0.,-0.866025403784443));
#8204=DIRECTION('center_axis',(-0.866025403784443,0.,-0.499999999999992));
#8205=DIRECTION('ref_axis',(-0.499999999999992,0.,0.866025403784443));
#8206=DIRECTION('',(0.866025403784443,0.,0.499999999999992));
#8207=DIRECTION('center_axis',(-0.866025403784443,0.,-0.499999999999992));
#8208=DIRECTION('ref_axis',(-0.499999999999992,0.,0.866025403784443));
#8209=DIRECTION('center_axis',(-0.612372435695796,0.707106781186546,-0.353553390593275));
#8210=DIRECTION('ref_axis',(-0.5,0.,0.866025403784438));
#8211=DIRECTION('center_axis',(-0.612372435695796,0.707106781186546,-0.353553390593275));
#8212=DIRECTION('ref_axis',(-0.755928946018453,-0.654653670707979,0.));
#8213=DIRECTION('center_axis',(-0.612372435695796,0.707106781186546,-0.353553390593275));
#8214=DIRECTION('ref_axis',(-0.755928946018453,-0.654653670707979,0.));
#8215=DIRECTION('center_axis',(-0.612372435695796,0.707106781186546,-0.353553390593275));
#8216=DIRECTION('ref_axis',(-0.755928946018453,-0.654653670707979,0.));
#8217=DIRECTION('',(-0.612372435695796,0.707106781186546,-0.353553390593275));
#8218=DIRECTION('center_axis',(0.,1.,0.));
#8219=DIRECTION('ref_axis',(0.,0.,1.));
#8220=DIRECTION('',(0.,1.,0.));
#8221=DIRECTION('center_axis',(-0.224143868042018,0.965925826289067,-0.129409522551263));
#8222=DIRECTION('ref_axis',(-0.974116947696296,-0.22604462437946,0.));
#8223=DIRECTION('',(-0.224143868042018,0.965925826289067,-0.129409522551263));
#8224=DIRECTION('center_axis',(-0.433012701892223,0.866025403784437,-0.250000000000002));
#8225=DIRECTION('ref_axis',(-0.894427190999914,-0.447213595499962,0.));
#8226=DIRECTION('',(-0.433012701892223,0.866025403784436,-0.250000000000002));
#8227=DIRECTION('center_axis',(-0.612372435695796,0.707106781186546,-0.353553390593275));
#8228=DIRECTION('ref_axis',(-0.755928946018453,-0.654653670707979,0.));
#8229=DIRECTION('',(-0.612372435695796,0.707106781186546,-0.353553390593275));
#8230=DIRECTION('center_axis',(0.433012701892215,0.499999999999992,-0.750000000000008));
#8231=DIRECTION('ref_axis',(-0.866025403784443,0.,-0.499999999999992));
#8232=DIRECTION('center_axis',(0.433012701892215,0.499999999999992,-0.750000000000008));
#8233=DIRECTION('ref_axis',(-0.649519052838319,0.750000000000008,0.125000000000006));
#8234=DIRECTION('center_axis',(-0.433012701892215,-0.499999999999992,0.750000000000008));
#8235=DIRECTION('ref_axis',(0.649519052838319,-0.750000000000008,-0.125000000000006));
#8236=DIRECTION('center_axis',(-0.433012701892215,-0.499999999999992,0.750000000000008));
#8237=DIRECTION('ref_axis',(0.649519052838319,-0.750000000000008,-0.125000000000006));
#8238=DIRECTION('',(0.433012701892215,0.499999999999992,-0.750000000000008));
#8239=DIRECTION('',(-0.433012701892199,-0.500000000000005,0.750000000000008));
#8240=DIRECTION('',(-0.433012701892214,-0.499999999999978,0.750000000000018));
#8241=DIRECTION('center_axis',(-0.433012701892211,0.500000000000004,0.750000000000002));
#8242=DIRECTION('ref_axis',(0.866025403784443,0.,0.499999999999992));
#8243=DIRECTION('center_axis',(-0.433012701892211,0.500000000000004,0.750000000000002));
#8244=DIRECTION('ref_axis',(-0.649519052838324,-0.750000000000002,0.125000000000015));
#8245=DIRECTION('center_axis',(0.433012701892211,-0.500000000000004,-0.750000000000002));
#8246=DIRECTION('ref_axis',(0.649519052838324,0.750000000000002,-0.125000000000015));
#8247=DIRECTION('center_axis',(0.433012701892211,-0.500000000000004,-0.750000000000002));
#8248=DIRECTION('ref_axis',(0.649519052838324,0.750000000000002,-0.125000000000015));
#8249=DIRECTION('',(-0.433012701892211,0.500000000000004,0.750000000000002));
#8250=DIRECTION('',(0.433012701892208,-0.499999999999987,-0.750000000000015));
#8251=DIRECTION('',(0.433012701892233,-0.50000000000002,-0.749999999999979));
#8252=DIRECTION('center_axis',(0.642402019910919,0.482962913144524,-0.595034847165548));
#8253=DIRECTION('ref_axis',(-0.679542161318994,0.,-0.733636456966194));
#8254=DIRECTION('center_axis',(0.642402019910919,0.482962913144524,-0.595034847165548));
#8255=DIRECTION('ref_axis',(0.510942898759438,0.308782699291242,0.802240985506049));
#8256=DIRECTION('center_axis',(-0.642402019910919,-0.482962913144524,0.595034847165548));
#8257=DIRECTION('ref_axis',(-0.510942898759438,-0.308782699291242,-0.802240985506049));
#8258=DIRECTION('center_axis',(-0.642402019910919,-0.482962913144524,0.595034847165548));
#8259=DIRECTION('ref_axis',(-0.510942898759438,-0.308782699291242,-0.802240985506049));
#8260=DIRECTION('',(0.642402019910919,0.482962913144524,-0.595034847165548));
#8261=DIRECTION('center_axis',(-0.194114283826876,0.482962913144539,0.853853892268062));
#8262=DIRECTION('ref_axis',(0.975118889534635,0.,0.221682546161714));
#8263=DIRECTION('center_axis',(-0.194114283826876,0.482962913144539,0.853853892268062));
#8264=DIRECTION('ref_axis',(0.706703285860956,-0.534827323670698,0.463174048936862));
#8265=DIRECTION('center_axis',(0.194114283826876,-0.482962913144539,-0.853853892268062));
#8266=DIRECTION('ref_axis',(-0.706703285860956,0.534827323670698,-0.463174048936862));
#8267=DIRECTION('center_axis',(0.194114283826876,-0.482962913144539,-0.853853892268062));
#8268=DIRECTION('ref_axis',(-0.706703285860956,0.534827323670698,-0.463174048936862));
#8269=DIRECTION('',(-0.194114283826876,0.482962913144539,0.853853892268062));
#8270=DIRECTION('center_axis',(0.808012701892221,0.433012701892207,-0.399519052838338));
#8271=DIRECTION('ref_axis',(-0.443226594010285,0.,-0.89640960858418));
#8272=DIRECTION('center_axis',(0.808012701892221,0.433012701892207,-0.399519052838338));
#8273=DIRECTION('ref_axis',(0.365367827064589,0.163691536870759,0.916357698556077));
#8274=DIRECTION('center_axis',(-0.808012701892221,-0.433012701892208,0.399519052838338));
#8275=DIRECTION('ref_axis',(-0.365367827064589,-0.163691536870759,-0.916357698556077));
#8276=DIRECTION('center_axis',(-0.808012701892221,-0.433012701892207,0.399519052838338));
#8277=DIRECTION('ref_axis',(-0.365367827064589,-0.163691536870759,-0.916357698556077));
#8278=DIRECTION('',(0.808012701892221,0.433012701892207,-0.399519052838338));
#8279=DIRECTION('center_axis',(0.058012701892234,0.433012701892226,0.899519052838325));
#8280=DIRECTION('ref_axis',(0.997926790235505,0.,-0.064359314246356));
#8281=DIRECTION('center_axis',(0.058012701892234,0.433012701892226,0.899519052838325));
#8282=DIRECTION('ref_axis',(0.752666161685325,-0.610905132370716,0.245537305306135));
#8283=DIRECTION('center_axis',(-0.0580127018922341,-0.433012701892225,-0.899519052838325));
#8284=DIRECTION('ref_axis',(-0.752666161685325,0.610905132370716,-0.245537305306135));
#8285=DIRECTION('center_axis',(-0.058012701892234,-0.433012701892226,-0.899519052838325));
#8286=DIRECTION('ref_axis',(-0.752666161685325,0.610905132370716,-0.245537305306135));
#8287=DIRECTION('',(0.058012701892234,0.433012701892226,0.899519052838325));
#8288=DIRECTION('center_axis',(0.918558653543694,0.353553390593261,-0.176776695296649));
#8289=DIRECTION('ref_axis',(-0.188982236504625,0.,-0.981980506061963));
#8290=DIRECTION('center_axis',(0.918558653543694,0.353553390593261,-0.176776695296649));
#8291=DIRECTION('ref_axis',(0.188982236504626,0.,0.981980506061964));
#8292=DIRECTION('center_axis',(-0.918558653543694,-0.353553390593261,0.176776695296649));
#8293=DIRECTION('ref_axis',(-0.188982236504626,-5.55111512312578E-17,-0.981980506061963));
#8294=DIRECTION('center_axis',(-0.918558653543694,-0.353553390593261,0.176776695296649));
#8295=DIRECTION('ref_axis',(-0.188982236504626,0.,-0.981980506061964));
#8296=DIRECTION('',(0.918558653543694,0.353553390593261,-0.176776695296649));
#8297=DIRECTION('center_axis',(0.30618621784791,0.353553390593282,0.883883476483177));
#8298=DIRECTION('ref_axis',(0.944911182523063,0.,-0.327326835354004));
#8299=DIRECTION('center_axis',(0.30618621784791,0.353553390593282,0.883883476483177));
#8300=DIRECTION('ref_axis',(0.755928946018457,-0.654653670707974,-7.66053886991358E-15));
#8301=DIRECTION('center_axis',(-0.30618621784791,-0.353553390593282,-0.883883476483177));
#8302=DIRECTION('ref_axis',(-0.755928946018457,0.654653670707974,7.60502771868232E-15));
#8303=DIRECTION('center_axis',(-0.30618621784791,-0.353553390593282,-0.883883476483177));
#8304=DIRECTION('ref_axis',(-0.755928946018457,0.654653670707974,7.66053886991358E-15));
#8305=DIRECTION('',(0.30618621784791,0.353553390593282,0.883883476483177));
#8306=DIRECTION('center_axis',(0.433012701892215,-0.499999999999992,-0.750000000000008));
#8307=DIRECTION('ref_axis',(0.649519052838319,0.750000000000008,-0.125000000000006));
#8308=DIRECTION('',(0.433012701892215,-0.499999999999992,-0.750000000000008));
#8309=DIRECTION('center_axis',(0.433012701892211,-0.500000000000004,-0.750000000000002));
#8310=DIRECTION('ref_axis',(0.,0.832050294337842,-0.554700196225231));
#8311=DIRECTION('center_axis',(-0.433012701892211,-0.500000000000004,0.750000000000002));
#8312=DIRECTION('ref_axis',(0.649519052838324,-0.750000000000002,-0.125000000000015));
#8313=DIRECTION('',(-0.433012701892211,-0.500000000000004,0.750000000000002));
#8314=DIRECTION('center_axis',(-0.433012701892215,-0.499999999999992,0.750000000000008));
#8315=DIRECTION('ref_axis',(0.,-0.832050294337851,-0.554700196225219));
#8316=DIRECTION('center_axis',(0.194114283826879,-0.482962913144528,-0.853853892268068));
#8317=DIRECTION('ref_axis',(-0.70670328586096,0.534827323670699,-0.463174048936855));
#8318=DIRECTION('',(0.194114283826879,-0.482962913144527,-0.853853892268068));
#8319=DIRECTION('center_axis',(0.194114283826876,-0.482962913144539,-0.853853892268062));
#8320=DIRECTION('ref_axis',(0.,0.87041002959648,-0.492327513326093));
#8321=DIRECTION('center_axis',(-0.642402019910915,-0.482962913144535,0.595034847165542));
#8322=DIRECTION('ref_axis',(-0.510942898759436,-0.308782699291236,-0.802240985506053));
#8323=DIRECTION('',(-0.642402019910915,-0.482962913144535,0.595034847165542));
#8324=DIRECTION('center_axis',(-0.642402019910919,-0.482962913144524,0.595034847165548));
#8325=DIRECTION('ref_axis',(0.679542161318994,0.,0.733636456966194));
#8326=DIRECTION('center_axis',(-0.0580127018922311,-0.433012701892215,-0.89951905283833));
#8327=DIRECTION('ref_axis',(-0.752666161685329,0.610905132370714,-0.245537305306127));
#8328=DIRECTION('',(-0.0580127018922311,-0.433012701892215,-0.89951905283833));
#8329=DIRECTION('center_axis',(-0.0580127018922341,-0.433012701892225,-0.899519052838325));
#8330=DIRECTION('ref_axis',(0.,0.901036538010451,-0.433743192649915));
#8331=DIRECTION('center_axis',(-0.808012701892218,-0.433012701892218,0.399519052838333));
#8332=DIRECTION('ref_axis',(-0.365367827064587,-0.163691536870751,-0.916357698556079));
#8333=DIRECTION('',(-0.808012701892218,-0.433012701892218,0.399519052838333));
#8334=DIRECTION('center_axis',(-0.808012701892221,-0.433012701892208,0.399519052838338));
#8335=DIRECTION('ref_axis',(0.472347490483135,-0.881412416655384,0.));
#8336=DIRECTION('center_axis',(-0.306186217847908,-0.353553390593273,-0.883883476483181));
#8337=DIRECTION('ref_axis',(-0.755928946018462,0.654653670707968,1.58761892521397E-14));
#8338=DIRECTION('',(-0.306186217847908,-0.353553390593273,-0.883883476483181));
#8339=DIRECTION('center_axis',(-0.30618621784791,-0.353553390593282,-0.883883476483177));
#8340=DIRECTION('ref_axis',(0.,0.928476690885255,-0.371390676354114));
#8341=DIRECTION('center_axis',(-0.918558653543692,-0.35355339059327,0.176776695296645));
#8342=DIRECTION('ref_axis',(-0.188982236504625,1.0547118733939E-14,-0.981980506061964));
#8343=DIRECTION('',(-0.918558653543692,-0.35355339059327,0.176776695296645));
#8344=DIRECTION('center_axis',(-0.918558653543694,-0.353553390593261,0.176776695296649));
#8345=DIRECTION('ref_axis',(0.359210604053538,-0.933256525257387,0.));
#8346=DIRECTION('center_axis',(-0.433012701892215,-0.499999999999992,0.750000000000008));
#8347=DIRECTION('ref_axis',(0.866025403784443,0.,0.499999999999992));
#8348=DIRECTION('center_axis',(-0.433012701892215,-0.499999999999992,0.750000000000008));
#8349=DIRECTION('ref_axis',(0.649519052838319,-0.750000000000008,-0.125000000000006));
#8350=DIRECTION('center_axis',(-0.433012701892215,-0.499999999999992,0.750000000000008));
#8351=DIRECTION('ref_axis',(0.649519052838319,-0.750000000000008,-0.125000000000006));
#8352=DIRECTION('',(-0.433012701892215,-0.499999999999992,0.750000000000008));
#8353=DIRECTION('center_axis',(0.433012701892211,-0.500000000000004,-0.750000000000002));
#8354=DIRECTION('ref_axis',(-0.866025403784443,0.,-0.499999999999992));
#8355=DIRECTION('center_axis',(0.433012701892211,-0.500000000000004,-0.750000000000002));
#8356=DIRECTION('ref_axis',(0.649519052838324,0.750000000000002,-0.125000000000015));
#8357=DIRECTION('center_axis',(0.433012701892211,-0.500000000000004,-0.750000000000002));
#8358=DIRECTION('ref_axis',(0.649519052838324,0.750000000000002,-0.125000000000015));
#8359=DIRECTION('',(0.433012701892211,-0.500000000000004,-0.750000000000002));
#8360=DIRECTION('center_axis',(-0.642402019910919,-0.482962913144524,0.595034847165548));
#8361=DIRECTION('ref_axis',(0.679542161318994,0.,0.733636456966194));
#8362=DIRECTION('center_axis',(-0.642402019910919,-0.482962913144524,0.595034847165548));
#8363=DIRECTION('ref_axis',(-0.510942898759438,-0.308782699291242,-0.802240985506049));
#8364=DIRECTION('center_axis',(-0.642402019910919,-0.482962913144524,0.595034847165548));
#8365=DIRECTION('ref_axis',(-0.510942898759438,-0.308782699291242,-0.802240985506049));
#8366=DIRECTION('',(-0.642402019910919,-0.482962913144524,0.595034847165548));
#8367=DIRECTION('center_axis',(0.194114283826876,-0.482962913144539,-0.853853892268062));
#8368=DIRECTION('ref_axis',(-0.975118889534635,0.,-0.221682546161714));
#8369=DIRECTION('center_axis',(0.194114283826876,-0.482962913144539,-0.853853892268062));
#8370=DIRECTION('ref_axis',(-0.706703285860956,0.534827323670698,-0.463174048936862));
#8371=DIRECTION('center_axis',(0.194114283826876,-0.482962913144539,-0.853853892268062));
#8372=DIRECTION('ref_axis',(-0.706703285860956,0.534827323670698,-0.463174048936862));
#8373=DIRECTION('',(0.194114283826876,-0.482962913144539,-0.853853892268062));
#8374=DIRECTION('center_axis',(-0.808012701892221,-0.433012701892208,0.399519052838338));
#8375=DIRECTION('ref_axis',(0.443226594010285,0.,0.89640960858418));
#8376=DIRECTION('center_axis',(-0.808012701892221,-0.433012701892208,0.399519052838338));
#8377=DIRECTION('ref_axis',(-0.365367827064589,-0.163691536870759,-0.916357698556077));
#8378=DIRECTION('center_axis',(-0.808012701892221,-0.433012701892207,0.399519052838338));
#8379=DIRECTION('ref_axis',(-0.365367827064589,-0.163691536870759,-0.916357698556077));
#8380=DIRECTION('',(-0.808012701892221,-0.433012701892207,0.399519052838338));
#8381=DIRECTION('center_axis',(-0.0580127018922341,-0.433012701892225,-0.899519052838325));
#8382=DIRECTION('ref_axis',(-0.997926790235505,0.,0.0643593142463562));
#8383=DIRECTION('center_axis',(-0.0580127018922341,-0.433012701892225,-0.899519052838325));
#8384=DIRECTION('ref_axis',(-0.752666161685325,0.610905132370716,-0.245537305306135));
#8385=DIRECTION('center_axis',(-0.0580127018922342,-0.433012701892225,-0.899519052838325));
#8386=DIRECTION('ref_axis',(-0.752666161685325,0.610905132370716,-0.245537305306135));
#8387=DIRECTION('',(-0.0580127018922342,-0.433012701892225,-0.899519052838325));
#8388=DIRECTION('center_axis',(-0.918558653543694,-0.353553390593261,0.176776695296649));
#8389=DIRECTION('ref_axis',(0.188982236504625,0.,0.981980506061963));
#8390=DIRECTION('center_axis',(-0.918558653543694,-0.353553390593261,0.176776695296649));
#8391=DIRECTION('ref_axis',(-0.188982236504626,-5.55111512312578E-17,-0.981980506061963));
#8392=DIRECTION('center_axis',(-0.918558653543694,-0.353553390593261,0.176776695296649));
#8393=DIRECTION('ref_axis',(-0.188982236504626,0.,-0.981980506061963));
#8394=DIRECTION('',(-0.918558653543694,-0.353553390593261,0.176776695296649));
#8395=DIRECTION('center_axis',(-0.30618621784791,-0.353553390593282,-0.883883476483177));
#8396=DIRECTION('ref_axis',(-0.944911182523063,0.,0.327326835354004));
#8397=DIRECTION('center_axis',(-0.30618621784791,-0.353553390593282,-0.883883476483177));
#8398=DIRECTION('ref_axis',(-0.755928946018457,0.654653670707974,7.60502771868232E-15));
#8399=DIRECTION('center_axis',(-0.306186217847911,-0.353553390593282,-0.883883476483177));
#8400=DIRECTION('ref_axis',(-0.755928946018457,0.654653670707974,7.66053886991358E-15));
#8401=DIRECTION('',(-0.30618621784791,-0.353553390593282,-0.883883476483177));
#8402=DIRECTION('center_axis',(-0.499999999999992,0.,0.866025403784443));
#8403=DIRECTION('ref_axis',(0.866025403784443,0.,0.499999999999992));
#8404=DIRECTION('',(0.866025403784443,0.,0.499999999999992));
#8405=DIRECTION('center_axis',(0.499999999999992,0.,-0.866025403784443));
#8406=DIRECTION('ref_axis',(-0.866025403784443,0.,-0.499999999999992));
#8407=DIRECTION('',(0.866025403784443,0.,0.499999999999992));
#8408=DIRECTION('center_axis',(-0.499999999999999,0.,0.866025403784439));
#8409=DIRECTION('ref_axis',(0.866025403784439,0.,0.499999999999999));
#8410=DIRECTION('',(0.,1.,0.));
#8411=DIRECTION('',(0.866025403784443,0.,0.499999999999992));
#8412=DIRECTION('center_axis',(0.499999999999999,0.,-0.866025403784439));
#8413=DIRECTION('ref_axis',(-0.866025403784439,0.,-0.499999999999999));
#8414=DIRECTION('',(0.866025403784443,0.,0.499999999999992));
#8415=DIRECTION('',(0.,1.,0.));
#8416=DIRECTION('center_axis',(0.866025403784443,0.,0.499999999999992));
#8417=DIRECTION('ref_axis',(0.499999999999992,0.,-0.866025403784443));
#8418=DIRECTION('center_axis',(0.249999999999998,0.866025403784436,-0.433012701892225));
#8419=DIRECTION('ref_axis',(-0.866025403784443,0.,-0.499999999999992));
#8420=DIRECTION('',(0.866025403784443,0.,0.499999999999992));
#8421=DIRECTION('center_axis',(-0.249999999999998,-0.866025403784436,0.433012701892225));
#8422=DIRECTION('ref_axis',(0.866025403784444,0.,0.499999999999991));
#8423=DIRECTION('',(0.866025403784443,0.,0.499999999999992));
#8424=DIRECTION('center_axis',(0.249999999999991,0.866025403784436,-0.433012701892229));
#8425=DIRECTION('ref_axis',(-0.866025403784452,0.,-0.499999999999977));
#8426=DIRECTION('',(0.433012701892214,-0.500000000000001,-0.750000000000002));
#8427=DIRECTION('',(0.866025403784443,0.,0.499999999999992));
#8428=DIRECTION('center_axis',(-0.249999999999991,-0.866025403784436,0.433012701892229));
#8429=DIRECTION('ref_axis',(0.866025403784451,0.,0.499999999999978));
#8430=DIRECTION('',(0.866025403784443,0.,0.499999999999992));
#8431=DIRECTION('',(0.433012701892241,-0.499999999999971,-0.750000000000007));
#8432=DIRECTION('center_axis',(0.866025403784443,0.,0.499999999999992));
#8433=DIRECTION('ref_axis',(0.499999999999992,0.,-0.866025403784443));
#8434=DIRECTION('center_axis',(0.249999999999992,-0.866025403784443,-0.433012701892215));
#8435=DIRECTION('ref_axis',(0.,0.447213595499952,-0.894427190999919));
#8436=DIRECTION('',(0.866025403784443,0.,0.499999999999992));
#8437=DIRECTION('center_axis',(-0.249999999999991,0.866025403784443,0.433012701892215));
#8438=DIRECTION('ref_axis',(0.,-0.447213595499952,0.894427190999919));
#8439=DIRECTION('',(0.866025403784443,0.,0.499999999999992));
#8440=DIRECTION('center_axis',(0.249999999999984,-0.866025403784443,-0.433012701892219));
#8441=DIRECTION('ref_axis',(0.,0.447213595499956,-0.894427190999917));
#8442=DIRECTION('',(-0.433012701892197,-0.499999999999982,0.750000000000025));
#8443=DIRECTION('',(0.866025403784443,0.,0.499999999999992));
#8444=DIRECTION('center_axis',(-0.249999999999985,0.866025403784443,0.433012701892219));
#8445=DIRECTION('ref_axis',(0.,-0.447213595499956,0.894427190999917));
#8446=DIRECTION('',(0.866025403784443,0.,0.499999999999992));
#8447=DIRECTION('',(-0.433012701892228,-0.49999999999999,0.750000000000002));
#8448=DIRECTION('center_axis',(0.866025403784443,0.,0.499999999999992));
#8449=DIRECTION('ref_axis',(0.499999999999992,0.,-0.866025403784443));
#8450=DIRECTION('center_axis',(-0.499999999999992,0.,0.866025403784443));
#8451=DIRECTION('ref_axis',(0.866025403784443,0.,0.499999999999992));
#8452=DIRECTION('',(0.866025403784442,0.,0.499999999999994));
#8453=DIRECTION('center_axis',(0.499999999999992,0.,-0.866025403784443));
#8454=DIRECTION('ref_axis',(-0.866025403784443,0.,-0.499999999999992));
#8455=DIRECTION('',(0.866025403784443,0.,0.499999999999992));
#8456=DIRECTION('center_axis',(0.,1.,0.));
#8457=DIRECTION('ref_axis',(0.,0.,1.));
#8458=DIRECTION('center_axis',(0.249999999999992,-0.866025403784443,-0.433012701892215));
#8459=DIRECTION('ref_axis',(0.,0.447213595499952,-0.894427190999919));
#8460=DIRECTION('',(0.866025403784443,0.,0.499999999999992));
#8461=DIRECTION('center_axis',(-0.249999999999992,0.866025403784443,0.433012701892215));
#8462=DIRECTION('ref_axis',(0.,-0.447213595499952,0.894427190999919));
#8463=DIRECTION('',(0.866025403784444,0.,0.499999999999991));
#8464=DIRECTION('center_axis',(-0.433012701892215,-0.499999999999992,0.750000000000008));
#8465=DIRECTION('ref_axis',(0.866025403784443,0.,0.499999999999992));
#8466=DIRECTION('center_axis',(0.249999999999998,0.866025403784436,-0.433012701892225));
#8467=DIRECTION('ref_axis',(-0.866025403784443,0.,-0.499999999999992));
#8468=DIRECTION('',(0.866025403784442,0.,0.499999999999994));
#8469=DIRECTION('center_axis',(-0.249999999999998,-0.866025403784436,0.433012701892225));
#8470=DIRECTION('ref_axis',(0.866025403784443,0.,0.499999999999992));
#8471=DIRECTION('',(0.866025403784442,0.,0.499999999999994));
#8472=DIRECTION('center_axis',(0.433012701892211,-0.500000000000004,-0.750000000000002));
#8473=DIRECTION('ref_axis',(-0.866025403784443,0.,-0.499999999999992));
#12317=CARTESIAN_POINT('',(0.,0.,0.));
#12318=CARTESIAN_POINT('Origin',(-69.7150450046476,109.,-52.2499999999992));
#12319=CARTESIAN_POINT('',(-57.0362860918569,101.937180526611,-60.2102546138697));
#12320=CARTESIAN_POINT('',(-60.5003877069947,101.937180526611,-62.2102546138697));
#12321=CARTESIAN_POINT('',(-60.5003877069947,101.937180526611,-62.2102546138697));
#12322=CARTESIAN_POINT('',(-63.4028671781572,123.991664350565,-49.1830127018903));
#12323=CARTESIAN_POINT('Origin',(-63.6528671781565,109.,-48.7499999999993));
#12324=CARTESIAN_POINT('',(-66.866968793295,123.991664350565,-51.1830127018903));
#12325=CARTESIAN_POINT('',(-66.866968793295,123.991664350565,-51.1830127018903));
#12326=CARTESIAN_POINT('Origin',(-67.1169687932943,109.,-50.7499999999993));
#12327=CARTESIAN_POINT('Origin',(-69.7150450046476,109.,-52.2499999999992));
#12328=CARTESIAN_POINT('',(-60.7503877069946,101.071155122826,-61.7772419119775));
#12329=CARTESIAN_POINT('',(-57.2862860918569,101.071155122826,-59.7772419119775));
#12330=CARTESIAN_POINT('',(-60.7503877069946,101.071155122826,-61.7772419119775));
#12331=CARTESIAN_POINT('',(-73.4835498795932,101.071155122824,-39.7227580880222));
#12332=CARTESIAN_POINT('Origin',(-67.1169687932943,109.,-50.7499999999993));
#12333=CARTESIAN_POINT('',(-70.0194482644555,101.071155122824,-37.7227580880222));
#12334=CARTESIAN_POINT('',(-73.4835498795932,101.071155122824,-39.7227580880221));
#12335=CARTESIAN_POINT('Origin',(-63.6528671781565,109.,-48.7499999999993));
#12336=CARTESIAN_POINT('Origin',(-119.078493020361,109.,-80.7499999999988));
#12337=CARTESIAN_POINT('',(-65.5747753124034,96.49269543419,-59.421157464004));
#12338=CARTESIAN_POINT('',(-73.855314696892,96.4926954341901,-45.0788425359943));
#12339=CARTESIAN_POINT('Origin',(-69.7150450046476,109.,-52.2499999999992));
#12340=CARTESIAN_POINT('',(-123.218762712605,96.4926954341901,-73.5788425359939));
#12341=CARTESIAN_POINT('',(-123.218762712605,96.4926954341901,-73.5788425359939));
#12342=CARTESIAN_POINT('',(-114.938223328117,96.49269543419,-87.9211574640035));
#12343=CARTESIAN_POINT('Origin',(-119.078493020361,109.,-80.7499999999988));
#12344=CARTESIAN_POINT('',(-114.938223328117,96.49269543419,-87.9211574640035));
#12345=CARTESIAN_POINT('Origin',(-119.078493020361,109.,-80.7499999999988));
#12346=CARTESIAN_POINT('',(-94.3860089394201,105.235685467736,-49.7275542973482));
#12347=CARTESIAN_POINT('',(-82.8207084929668,105.235685467736,-43.0503249713298));
#12348=CARTESIAN_POINT('',(-94.3860089394201,105.235685467737,-49.7275542973482));
#12349=CARTESIAN_POINT('',(-91.0176401746589,103.250749366077,-48.5513043322017));
#12350=CARTESIAN_POINT('Ctrl Pts',(-91.0176401746589,103.250749366077,-48.5513043322017));
#12351=CARTESIAN_POINT('Ctrl Pts',(-91.2361059276669,103.557750420993,-48.5303294493383));
#12352=CARTESIAN_POINT('Ctrl Pts',(-91.4832335600058,103.842139746856,-48.5508334265686));
#12353=CARTESIAN_POINT('Ctrl Pts',(-92.1066673879442,104.430592760333,-48.6750977465524));
#12354=CARTESIAN_POINT('Ctrl Pts',(-92.5431699718694,104.735168552794,-48.8223964645982));
#12355=CARTESIAN_POINT('Ctrl Pts',(-93.461912716518,105.137985045737,-49.2219363914119));
#12356=CARTESIAN_POINT('Ctrl Pts',(-93.9449426785634,105.235685467736,-49.4729045729122));
#12357=CARTESIAN_POINT('Ctrl Pts',(-94.3860089394201,105.235685467736,-49.7275542973483));
#12358=CARTESIAN_POINT('',(-92.3860089394197,98.3074822374609,-53.1916559124865));
#12359=CARTESIAN_POINT('Ctrl Pts',(-92.3860089394197,98.307482237461,-53.1916559124864));
#12360=CARTESIAN_POINT('Ctrl Pts',(-91.944942678563,98.307482237461,-52.9370061880504));
#12361=CARTESIAN_POINT('Ctrl Pts',(-91.5102607802988,98.3772644212952,-52.6022967036335));
#12362=CARTESIAN_POINT('Ctrl Pts',(-90.7942826050959,98.676845000861,-51.8515582405649));
#12363=CARTESIAN_POINT('Ctrl Pts',(-90.5123369230427,98.9076700218055,-51.4365591158164));
#12364=CARTESIAN_POINT('Ctrl Pts',(-90.1413389560881,99.4578375470661,-50.6726253387866));
#12365=CARTESIAN_POINT('Ctrl Pts',(-90.0255053791506,99.8112989429842,-50.2740223286365));
#12366=CARTESIAN_POINT('Ctrl Pts',(-89.9729277960154,100.614428273412,-49.573341944019));
#12367=CARTESIAN_POINT('Ctrl Pts',(-90.0353007740436,101.064744995698,-49.2720751413297));
#12368=CARTESIAN_POINT('Ctrl Pts',(-90.2865953679429,101.9352550043,-48.8368201370289));
#12369=CARTESIAN_POINT('Ctrl Pts',(-90.4922380489042,102.413371759201,-48.6738702011243));
#12370=CARTESIAN_POINT('Ctrl Pts',(-90.8440070426079,102.99654996933,-48.5751774684912));
#12371=CARTESIAN_POINT('Ctrl Pts',(-90.9285040512729,103.125489990024,-48.559862285662));
#12372=CARTESIAN_POINT('Ctrl Pts',(-91.0176401746589,103.250749366077,-48.5513043322017));
#12373=CARTESIAN_POINT('',(-80.8207084929665,98.3074822374608,-46.5144265864682));
#12374=CARTESIAN_POINT('',(-92.3860089394198,98.3074822374611,-53.1916559124864));
#12375=CARTESIAN_POINT('',(-84.4784050214276,104.702740240336,-44.1791103605043));
#12376=CARTESIAN_POINT('Ctrl Pts',(-84.4784050214273,104.702740240336,-44.179110360504));
#12377=CARTESIAN_POINT('Ctrl Pts',(-84.719910157753,104.526945752297,-44.3792409314819));
#12378=CARTESIAN_POINT('Ctrl Pts',(-84.9292227283709,104.313493521274,-44.5780840276366));
#12379=CARTESIAN_POINT('Ctrl Pts',(-85.3433081511931,103.743726568118,-45.0453786543482));
#12380=CARTESIAN_POINT('Ctrl Pts',(-85.5286602574863,103.319666529342,-45.3392616445606));
#12381=CARTESIAN_POINT('Ctrl Pts',(-85.6804888744289,102.416155145618,-45.8942563092267));
#12382=CARTESIAN_POINT('Ctrl Pts',(-85.6462202716666,101.937209973523,-46.1563950132377));
#12383=CARTESIAN_POINT('Ctrl Pts',(-85.3937969757602,101.062790026475,-46.5936049867616));
#12384=CARTESIAN_POINT('Ctrl Pts',(-85.1596379659028,100.611874672147,-46.7963965459624));
#12385=CARTESIAN_POINT('Ctrl Pts',(-84.5153961509797,99.8096167014324,-47.0942865585158));
#12386=CARTESIAN_POINT('Ctrl Pts',(-84.1059621410022,99.4574342557325,-47.1885248105415));
#12387=CARTESIAN_POINT('Ctrl Pts',(-83.2575101221815,98.9126166677475,-47.2430172368065));
#12388=CARTESIAN_POINT('Ctrl Pts',(-82.7609372275344,98.6829050367047,-47.2068324926174));
#12389=CARTESIAN_POINT('Ctrl Pts',(-81.7609021788356,98.3807025943171,-46.9694819795316));
#12390=CARTESIAN_POINT('Ctrl Pts',(-81.2579982865691,98.3074822374608,-46.7668959665184));
#12391=CARTESIAN_POINT('Ctrl Pts',(-80.8207084929665,98.3074822374608,-46.5144265864681));
#12392=CARTESIAN_POINT('Ctrl Pts',(-82.8207084929668,105.235685467736,-43.0503249713298));
#12393=CARTESIAN_POINT('Ctrl Pts',(-83.2579982865694,105.235685467736,-43.3027943513801));
#12394=CARTESIAN_POINT('Ctrl Pts',(-83.7101950061769,105.133251025885,-43.5932077637468));
#12395=CARTESIAN_POINT('Ctrl Pts',(-84.2375848518395,104.864030249166,-43.985328869011));
#12396=CARTESIAN_POINT('Ctrl Pts',(-84.3616836412502,104.787703134226,-44.0823856414543));
#12397=CARTESIAN_POINT('Ctrl Pts',(-84.4784050214273,104.702740240336,-44.179110360504));
#12398=CARTESIAN_POINT('Origin',(-119.078493020361,109.,-80.7499999999988));
#12399=CARTESIAN_POINT('',(-105.931810542547,105.235685467737,-56.3935259609235));
#12400=CARTESIAN_POINT('',(-105.931810542547,105.235685467737,-56.3935259609236));
#12401=CARTESIAN_POINT('',(-102.208219994794,103.102717662028,-55.0841964154936));
#12402=CARTESIAN_POINT('Ctrl Pts',(-102.208219994794,103.102717662026,-55.0841964154936));
#12403=CARTESIAN_POINT('Ctrl Pts',(-102.449021592923,103.452288080539,-55.0506293513879));
#12404=CARTESIAN_POINT('Ctrl Pts',(-102.730142130046,103.775612080798,-55.0719387240821));
#12405=CARTESIAN_POINT('Ctrl Pts',(-103.427690853637,104.41668799164,-55.2155771708353));
#12406=CARTESIAN_POINT('Ctrl Pts',(-103.909507673844,104.73291730259,-55.385468864601));
#12407=CARTESIAN_POINT('Ctrl Pts',(-104.920531073176,105.142197830513,-55.8362211929756));
#12408=CARTESIAN_POINT('Ctrl Pts',(-105.450263434612,105.235685467736,-56.1155046085297));
#12409=CARTESIAN_POINT('Ctrl Pts',(-105.931810542547,105.235685467736,-56.3935259609236));
#12410=CARTESIAN_POINT('',(-103.931810542547,98.307482237461,-59.8576275760617));
#12411=CARTESIAN_POINT('Ctrl Pts',(-103.931810542547,98.3074822374611,-59.8576275760617));
#12412=CARTESIAN_POINT('Ctrl Pts',(-103.450263434612,98.3074822374611,-59.5796062236677));
#12413=CARTESIAN_POINT('Ctrl Pts',(-102.966762319561,98.3741443355121,-59.2202479404765));
#12414=CARTESIAN_POINT('Ctrl Pts',(-102.161749770577,98.6785063270139,-58.4126743523891));
#12415=CARTESIAN_POINT('Ctrl Pts',(-101.840308730574,98.9178350152992,-57.9650036590062));
#12416=CARTESIAN_POINT('Ctrl Pts',(-101.440098436538,99.4841271059821,-57.1713087801904));
#12417=CARTESIAN_POINT('Ctrl Pts',(-101.317391802105,99.8312991080725,-56.7758910574572));
#12418=CARTESIAN_POINT('Ctrl Pts',(-101.255012945074,100.623349028226,-56.0804534046886));
#12419=CARTESIAN_POINT('Ctrl Pts',(-101.314116564966,101.068801289505,-55.7811982784879));
#12420=CARTESIAN_POINT('Ctrl Pts',(-101.563069256545,101.931198710494,-55.3499995679935));
#12421=CARTESIAN_POINT('Ctrl Pts',(-101.769030711735,102.403958803925,-55.1901485168392));
#12422=CARTESIAN_POINT('Ctrl Pts',(-102.095779742704,102.93486881927,-55.1031827978842));
#12423=CARTESIAN_POINT('Ctrl Pts',(-102.150902897407,103.019510732018,-55.0921862573272));
#12424=CARTESIAN_POINT('Ctrl Pts',(-102.208219994794,103.102717662026,-55.0841964154936));
#12425=CARTESIAN_POINT('',(-103.931810542547,98.3074822374611,-59.8576275760617));
#12426=CARTESIAN_POINT('Ctrl Pts',(-94.3860089394201,105.235685467736,-49.7275542973483));
#12427=CARTESIAN_POINT('Ctrl Pts',(-94.8437110509037,105.235685467736,-49.991808734622));
#12428=CARTESIAN_POINT('Ctrl Pts',(-95.3183294965658,105.131719766023,-50.2956435885911));
#12429=CARTESIAN_POINT('Ctrl Pts',(-96.1649446403336,104.726122671488,-50.9165050382747));
#12430=CARTESIAN_POINT('Ctrl Pts',(-96.5365223340826,104.425439262705,-51.2347212917227));
#12431=CARTESIAN_POINT('Ctrl Pts',(-97.079067270285,103.751330105903,-51.8179767152385));
#12432=CARTESIAN_POINT('Ctrl Pts',(-97.2914477713889,103.33295780308,-52.124268380383));
#12433=CARTESIAN_POINT('Ctrl Pts',(-97.4838471817179,102.430163538116,-52.7010684635898));
#12434=CARTESIAN_POINT('Ctrl Pts',(-97.4623083504636,101.946025606973,-52.9725395573328));
#12435=CARTESIAN_POINT('Ctrl Pts',(-97.2047953462119,101.053974393026,-53.4185651643064));
#12436=CARTESIAN_POINT('Ctrl Pts',(-96.9552287340129,100.59897551963,-53.616662472833));
#12437=CARTESIAN_POINT('Ctrl Pts',(-96.2710769848093,99.7982897132515,-53.8916024252977));
#12438=CARTESIAN_POINT('Ctrl Pts',(-95.8377694343555,99.451348267594,-53.9679676343933));
#12439=CARTESIAN_POINT('Ctrl Pts',(-94.9448662844064,98.9117809702792,-53.991550437936));
#12440=CARTESIAN_POINT('Ctrl Pts',(-94.4206402272791,98.683674936935,-53.9377289055515));
#12441=CARTESIAN_POINT('Ctrl Pts',(-93.3698028357836,98.3818254132703,-53.670590764968));
#12442=CARTESIAN_POINT('Ctrl Pts',(-92.8437110509033,98.307482237461,-53.4559103497602));
#12443=CARTESIAN_POINT('Ctrl Pts',(-92.3860089394197,98.307482237461,-53.1916559124864));
#12444=CARTESIAN_POINT('Origin',(-119.078493020361,109.,-80.7499999999988));
#12445=CARTESIAN_POINT('',(-117.424340315019,105.235685467737,-63.0287411187298));
#12446=CARTESIAN_POINT('',(-117.424340315019,105.235685467737,-63.0287411187298));
#12447=CARTESIAN_POINT('',(-112.873099678569,102.847499823892,-61.3708278876974));
#12448=CARTESIAN_POINT('Ctrl Pts',(-112.873099678569,102.847499823892,-61.3708278876974));
#12449=CARTESIAN_POINT('Ctrl Pts',(-112.885263071986,102.865530125643,-61.3684870415431));
#12450=CARTESIAN_POINT('Ctrl Pts',(-112.897548248638,102.883504310233,-61.366295141775));
#12451=CARTESIAN_POINT('Ctrl Pts',(-113.223445655223,103.354153784421,-61.312605698808));
#12452=CARTESIAN_POINT('Ctrl Pts',(-113.617943081627,103.765699546249,-61.3609453836262));
#12453=CARTESIAN_POINT('Ctrl Pts',(-114.51341914509,104.46875863804,-61.596335766007));
#12454=CARTESIAN_POINT('Ctrl Pts',(-115.084650741731,104.772419738951,-61.8242044014969));
#12455=CARTESIAN_POINT('Ctrl Pts',(-116.26458534071,105.155153282331,-62.3819677418281));
#12456=CARTESIAN_POINT('Ctrl Pts',(-116.873387883958,105.235685467737,-62.7106485843461));
#12457=CARTESIAN_POINT('Ctrl Pts',(-117.424340315019,105.235685467736,-63.0287411187299));
#12458=CARTESIAN_POINT('',(-115.424340315019,98.3074822374612,-66.4928427338677));
#12459=CARTESIAN_POINT('Ctrl Pts',(-115.424340315019,98.3074822374612,-66.4928427338678));
#12460=CARTESIAN_POINT('Ctrl Pts',(-114.873387883957,98.3074822374612,-66.1747501994839));
#12461=CARTESIAN_POINT('Ctrl Pts',(-114.304395627967,98.3648569324462,-65.7771159167707));
#12462=CARTESIAN_POINT('Ctrl Pts',(-113.316922034078,98.6488278676478,-64.8860003371488));
#12463=CARTESIAN_POINT('Ctrl Pts',(-112.899248494017,98.8771074785532,-64.3921613457507));
#12464=CARTESIAN_POINT('Ctrl Pts',(-112.369176942676,99.4398467473837,-63.5238717830588));
#12465=CARTESIAN_POINT('Ctrl Pts',(-112.191730388089,99.7801872611806,-63.0995889604281));
#12466=CARTESIAN_POINT('Ctrl Pts',(-112.057561335007,100.581884791004,-62.3492963885222));
#12467=CARTESIAN_POINT('Ctrl Pts',(-112.099359165682,101.044133890221,-62.0245059301422));
#12468=CARTESIAN_POINT('Ctrl Pts',(-112.357346552702,101.937828414283,-61.5776586681113));
#12469=CARTESIAN_POINT('Ctrl Pts',(-112.577858013516,102.409850877713,-61.4276471726289));
#12470=CARTESIAN_POINT('Ctrl Pts',(-112.873099678569,102.847499823891,-61.3708278876975));
#12471=CARTESIAN_POINT('',(-115.424340315019,98.3074822374611,-66.4928427338679));
#12472=CARTESIAN_POINT('Ctrl Pts',(-105.931810542547,105.235685467736,-56.3935259609236));
#12473=CARTESIAN_POINT('Ctrl Pts',(-106.441097653729,105.235685467736,-56.687563011659));
#12474=CARTESIAN_POINT('Ctrl Pts',(-106.974640486628,105.132960205187,-57.0250658019486));
#12475=CARTESIAN_POINT('Ctrl Pts',(-107.947581410815,104.730808636537,-57.7176366639949));
#12476=CARTESIAN_POINT('Ctrl Pts',(-108.386686426508,104.432320373104,-58.0736604657704));
#12477=CARTESIAN_POINT('Ctrl Pts',(-109.030432576161,103.765790736202,-58.7123084319066));
#12478=CARTESIAN_POINT('Ctrl Pts',(-109.294438065739,103.359086193815,-59.0420063444297));
#12479=CARTESIAN_POINT('Ctrl Pts',(-109.56709842014,102.458977333711,-59.6612621436709));
#12480=CARTESIAN_POINT('Ctrl Pts',(-109.572926265459,101.965344390994,-59.9517288812603));
#12481=CARTESIAN_POINT('Ctrl Pts',(-109.304259556052,101.034655609004,-60.4170732722551));
#12482=CARTESIAN_POINT('Ctrl Pts',(-109.022522963702,100.572512615502,-60.6044945027757));
#12483=CARTESIAN_POINT('Ctrl Pts',(-108.260113770694,99.7760817327768,-60.8335085749491));
#12484=CARTESIAN_POINT('Ctrl Pts',(-107.781619042588,99.4397737575475,-60.8753169212342));
#12485=CARTESIAN_POINT('Ctrl Pts',(-106.791454021988,98.9062732240887,-60.8366840402783));
#12486=CARTESIAN_POINT('Ctrl Pts',(-106.200906509653,98.6801492903,-60.7429663371135));
#12487=CARTESIAN_POINT('Ctrl Pts',(-105.025500473564,98.3809411378044,-60.40107533564));
#12488=CARTESIAN_POINT('Ctrl Pts',(-104.441097653728,98.3074822374611,-60.1516646267969));
#12489=CARTESIAN_POINT('Ctrl Pts',(-103.931810542547,98.3074822374611,-59.8576275760616));
#12490=CARTESIAN_POINT('Origin',(-119.078493020361,109.,-80.7499999999988));
#12491=CARTESIAN_POINT('',(-118.78998649473,98.3074822374612,-68.4359994617213));
#12492=CARTESIAN_POINT('',(-118.78998649473,98.3074822374611,-68.4359994617214));
#12493=CARTESIAN_POINT('Ctrl Pts',(-117.424340315019,105.235685467736,-63.0287411187299));
#12494=CARTESIAN_POINT('Ctrl Pts',(-118.104455067791,105.235685467737,-63.4214055543222));
#12495=CARTESIAN_POINT('Ctrl Pts',(-118.823383370921,105.115025708115,-63.8707727019096));
#12496=CARTESIAN_POINT('Ctrl Pts',(-120.152211057545,104.638615075121,-64.7952439254207));
#12497=CARTESIAN_POINT('Ctrl Pts',(-120.762708154872,104.285378551405,-65.27078272247));
#12498=CARTESIAN_POINT('Ctrl Pts',(-121.530321038309,103.561110088859,-66.0199577490771));
#12499=CARTESIAN_POINT('Ctrl Pts',(-121.807474740758,103.201357059968,-66.343360523086));
#12500=CARTESIAN_POINT('Ctrl Pts',(-122.043414724861,102.594072465734,-66.7981024939494));
#12501=CARTESIAN_POINT('Ctrl Pts',(-122.092678493038,102.380375656682,-66.945003657385));
#12502=CARTESIAN_POINT('Ctrl Pts',(-122.117297884372,101.943528113597,-67.2175789887018));
#12503=CARTESIAN_POINT('Ctrl Pts',(-122.092529257229,101.720365047742,-67.3432446008741));
#12504=CARTESIAN_POINT('Ctrl Pts',(-121.965301437595,101.279634952257,-67.5636096486164));
#12505=CARTESIAN_POINT('Ctrl Pts',(-121.863134141106,101.063079080039,-67.6578035054809));
#12506=CARTESIAN_POINT('Ctrl Pts',(-121.5934173484,100.650884319169,-67.8097493261416));
#12507=CARTESIAN_POINT('Ctrl Pts',(-121.425973083727,100.45519187943,-67.8675427871017));
#12508=CARTESIAN_POINT('Ctrl Pts',(-120.858109129937,99.9126581141667,-67.9877099959866));
#12509=CARTESIAN_POINT('Ctrl Pts',(-120.389803254753,99.6102405927516,-67.9953924971306));
#12510=CARTESIAN_POINT('Ctrl Pts',(-119.242323386653,99.0186112201875,-67.9041663880787));
#12511=CARTESIAN_POINT('Ctrl Pts',(-118.452225355267,98.7496918581534,-67.7397055339048));
#12512=CARTESIAN_POINT('Ctrl Pts',(-116.883055382911,98.393532390957,-67.231519360489));
#12513=CARTESIAN_POINT('Ctrl Pts',(-116.10445506779,98.3074822374612,-66.8855071694601));
#12514=CARTESIAN_POINT('Ctrl Pts',(-115.424340315019,98.3074822374612,-66.4928427338678));
#12515=CARTESIAN_POINT('',(-120.78998649473,105.235685467737,-64.9718978465832));
#12516=CARTESIAN_POINT('',(-120.78998649473,105.235685467737,-64.9718978465831));
#12517=CARTESIAN_POINT('Ctrl Pts',(-118.78998649473,98.3074822374612,-68.4359994617213));
#12518=CARTESIAN_POINT('Ctrl Pts',(-118.918348276834,98.3074822374612,-68.5101091711724));
#12519=CARTESIAN_POINT('Ctrl Pts',(-119.051966028522,98.319606062948,-68.5729797213706));
#12520=CARTESIAN_POINT('Ctrl Pts',(-119.390180292013,98.3776312711511,-68.7006060360938));
#12521=CARTESIAN_POINT('Ctrl Pts',(-119.594844068455,98.4360499331429,-68.7509667466566));
#12522=CARTESIAN_POINT('Ctrl Pts',(-120.108561068232,98.6351217911646,-68.822841039124));
#12523=CARTESIAN_POINT('Ctrl Pts',(-120.410333239601,98.8023575570841,-68.8132768624661));
#12524=CARTESIAN_POINT('Ctrl Pts',(-121.095658711484,99.2862798538955,-68.7087637376292));
#12525=CARTESIAN_POINT('Ctrl Pts',(-121.453647702316,99.6436546824008,-68.5719722406892));
#12526=CARTESIAN_POINT('Ctrl Pts',(-121.95322023847,100.313709548206,-68.2828712619504));
#12527=CARTESIAN_POINT('Ctrl Pts',(-122.13026373805,100.619480486203,-68.1403943115824));
#12528=CARTESIAN_POINT('Ctrl Pts',(-122.350414930589,101.118875846441,-67.8997101912188));
#12529=CARTESIAN_POINT('Ctrl Pts',(-122.419254299142,101.308117977183,-67.8067240343058));
#12530=CARTESIAN_POINT('Ctrl Pts',(-122.529732701345,101.690626616667,-67.6154765320548));
#12531=CARTESIAN_POINT('Ctrl Pts',(-122.571615353665,101.884694244957,-67.5168156573903));
#12532=CARTESIAN_POINT('Ctrl Pts',(-122.647401154913,102.409372784178,-67.2455011686517));
#12533=CARTESIAN_POINT('Ctrl Pts',(-122.655932486104,102.745023337843,-67.0673187398412));
#12534=CARTESIAN_POINT('Ctrl Pts',(-122.572273917842,103.513663673561,-66.6372167411127));
#12535=CARTESIAN_POINT('Ctrl Pts',(-122.443353045988,103.95119638048,-66.3765548091624));
#12536=CARTESIAN_POINT('Ctrl Pts',(-122.075417244245,104.56927639081,-65.9299074078767));
#12537=CARTESIAN_POINT('Ctrl Pts',(-121.885875205944,104.790787749988,-65.7451136026938));
#12538=CARTESIAN_POINT('Ctrl Pts',(-121.506987477856,105.058995953627,-65.4396037944961));
#12539=CARTESIAN_POINT('Ctrl Pts',(-121.342237738227,105.139116769073,-65.3199491226463));
#12540=CARTESIAN_POINT('Ctrl Pts',(-121.043690674034,105.218909586375,-65.1233635722866));
#12541=CARTESIAN_POINT('Ctrl Pts',(-120.918381560469,105.235685467737,-65.0460267723497));
#12542=CARTESIAN_POINT('Ctrl Pts',(-120.78998649473,105.235685467737,-64.9718978465831));
#12543=CARTESIAN_POINT('Origin',(-119.078493020361,109.,-80.7499999999988));
#12544=CARTESIAN_POINT('',(-66.3693581073396,122.42480974691,-58.0448996923544));
#12545=CARTESIAN_POINT('',(-62.2290884150953,108.0824948189,-65.2160571563592));
#12546=CARTESIAN_POINT('Origin',(-69.7150450046476,109.,-52.2499999999992));
#12547=CARTESIAN_POINT('',(-111.592536430809,108.0824948189,-93.7160571563587));
#12548=CARTESIAN_POINT('',(-111.592536430809,108.0824948189,-93.7160571563587));
#12549=CARTESIAN_POINT('',(-115.732806123053,122.42480974691,-86.5448996923539));
#12550=CARTESIAN_POINT('Origin',(-119.078493020361,109.,-80.7499999999988));
#12551=CARTESIAN_POINT('',(-115.732806123053,122.42480974691,-86.5448996923539));
#12552=CARTESIAN_POINT('Origin',(-119.078493020361,109.,-80.7499999999988));
#12553=CARTESIAN_POINT('',(-81.8660249138711,98.3074822374625,-71.4128027395503));
#12554=CARTESIAN_POINT('',(-70.3007244674178,98.3074822374627,-64.7355734135318));
#12555=CARTESIAN_POINT('',(-81.8660249138712,98.3074822374623,-71.4128027395501));
#12556=CARTESIAN_POINT('',(-78.1372951281693,99.8763092742309,-70.8607163717404));
#12557=CARTESIAN_POINT('Ctrl Pts',(-78.1372951281693,99.8763092742309,-70.8607163717404));
#12558=CARTESIAN_POINT('Ctrl Pts',(-78.3931479940217,99.6124791386442,-70.7749851098822));
#12559=CARTESIAN_POINT('Ctrl Pts',(-78.6840646784847,99.3786530548441,-70.7196442240182));
#12560=CARTESIAN_POINT('Ctrl Pts',(-79.4092304936657,98.9076700218071,-70.6677035733428));
#12561=CARTESIAN_POINT('Ctrl Pts',(-79.9096031192728,98.6768450008626,-70.704376134114));
#12562=CARTESIAN_POINT('Ctrl Pts',(-80.9177507874897,98.3772644212968,-70.9490621908606));
#12563=CARTESIAN_POINT('Ctrl Pts',(-81.4249586530144,98.3074822374626,-71.1581530151143));
#12564=CARTESIAN_POINT('Ctrl Pts',(-81.8660249138711,98.3074822374626,-71.4128027395504));
#12565=CARTESIAN_POINT('',(-79.8660249138713,105.235685467738,-74.8769043546876));
#12566=CARTESIAN_POINT('Ctrl Pts',(-79.8660249138713,105.235685467738,-74.8769043546876));
#12567=CARTESIAN_POINT('Ctrl Pts',(-79.4249586530146,105.235685467738,-74.6222546302515));
#12568=CARTESIAN_POINT('Ctrl Pts',(-78.966098851271,105.13798504574,-74.3294225030814));
#12569=CARTESIAN_POINT('Ctrl Pts',(-78.1607157524998,104.735168552796,-73.7335379100799));
#12570=CARTESIAN_POINT('Ctrl Pts',(-77.8149000287647,104.430592760335,-73.4291649426061));
#12571=CARTESIAN_POINT('Ctrl Pts',(-77.3250662827369,103.743205497,-72.8710607726881));
#12572=CARTESIAN_POINT('Ctrl Pts',(-77.1468233216009,103.317679951548,-72.580553986839));
#12573=CARTESIAN_POINT('Ctrl Pts',(-77.0066222737195,102.413371759203,-72.0316418950969));
#12574=CARTESIAN_POINT('Ctrl Pts',(-77.0449197172773,101.935255004302,-71.7720751413298));
#12575=CARTESIAN_POINT('Ctrl Pts',(-77.2962143111765,101.0647449957,-71.3368201370292));
#12576=CARTESIAN_POINT('Ctrl Pts',(-77.5259325266081,100.614428273414,-71.1321701522025));
#12577=CARTESIAN_POINT('Ctrl Pts',(-77.9342089099037,100.096499176469,-70.9356037497933));
#12578=CARTESIAN_POINT('Ctrl Pts',(-78.0329047040169,99.9839545009761,-70.895695549162));
#12579=CARTESIAN_POINT('Ctrl Pts',(-78.1372951281693,99.8763092742309,-70.8607163717404));
#12580=CARTESIAN_POINT('',(-68.3007244674181,105.235685467739,-68.1996750286692));
#12581=CARTESIAN_POINT('',(-79.8660249138713,105.235685467738,-74.8769043546876));
#12582=CARTESIAN_POINT('',(-71.8391803616632,98.7027402403375,-66.0708896394943));
#12583=CARTESIAN_POINT('Ctrl Pts',(-71.8391803616628,98.7027402403373,-66.070889639494));
#12584=CARTESIAN_POINT('Ctrl Pts',(-72.0439884445282,98.8361606209892,-66.3345813715533));
#12585=CARTESIAN_POINT('Ctrl Pts',(-72.2115336533623,99.001384056873,-66.6057676604154));
#12586=CARTESIAN_POINT('Ctrl Pts',(-72.5271374781293,99.4574342557344,-67.2436374185692));
#12587=CARTESIAN_POINT('Ctrl Pts',(-72.6502417628557,99.8096167014344,-67.645336798396));
#12588=CARTESIAN_POINT('Ctrl Pts',(-72.7143823519123,100.611874672149,-68.3522115825761));
#12589=CARTESIAN_POINT('Ctrl Pts',(-72.6558392149002,101.062790026477,-68.6563950132379));
#12590=CARTESIAN_POINT('Ctrl Pts',(-72.4034159189938,101.937209973525,-69.0936049867617));
#12591=CARTESIAN_POINT('Ctrl Pts',(-72.1935314433864,102.41615514562,-69.2543518193115));
#12592=CARTESIAN_POINT('Ctrl Pts',(-71.6369776563495,103.319666529344,-69.4003617123507));
#12593=CARTESIAN_POINT('Ctrl Pts',(-71.2897914679388,103.743726568121,-69.3867835747619));
#12594=CARTESIAN_POINT('Ctrl Pts',(-70.5589898894586,104.424395182907,-69.2374994608244));
#12595=CARTESIAN_POINT('Ctrl Pts',(-70.1256610955174,104.727134811084,-69.0917727209338));
#12596=CARTESIAN_POINT('Ctrl Pts',(-69.2156180135337,105.133251025888,-68.6985515492242));
#12597=CARTESIAN_POINT('Ctrl Pts',(-68.7380142610207,105.235685467739,-68.4521444087194));
#12598=CARTESIAN_POINT('Ctrl Pts',(-68.3007244674181,105.235685467739,-68.1996750286692));
#12599=CARTESIAN_POINT('Ctrl Pts',(-70.3007244674178,98.3074822374626,-64.7355734135318));
#12600=CARTESIAN_POINT('Ctrl Pts',(-70.7380142610204,98.3074822374626,-64.9880427935821));
#12601=CARTESIAN_POINT('Ctrl Pts',(-71.1649108408744,98.3807025943189,-65.3222773334404));
#12602=CARTESIAN_POINT('Ctrl Pts',(-71.63264360737,98.5810373096057,-65.817727530853));
#12603=CARTESIAN_POINT('Ctrl Pts',(-71.7401949633927,98.6382570943041,-65.9434452986592));
#12604=CARTESIAN_POINT('Ctrl Pts',(-71.8391803616628,98.7027402403373,-66.070889639494));
#12605=CARTESIAN_POINT('Origin',(-119.078493020361,109.,-80.7499999999988));
#12606=CARTESIAN_POINT('',(-93.4118265169985,98.3074822374623,-78.0787744031255));
#12607=CARTESIAN_POINT('',(-93.4118265169985,98.3074822374623,-78.0787744031255));
#12608=CARTESIAN_POINT('',(-89.310545785853,100.004330985067,-77.4236234448516));
#12609=CARTESIAN_POINT('Ctrl Pts',(-89.3105457858516,100.004330985068,-77.4236234448524));
#12610=CARTESIAN_POINT('Ctrl Pts',(-89.5906127684196,99.7001003271067,-77.3220467399197));
#12611=CARTESIAN_POINT('Ctrl Pts',(-89.9201573466291,99.432691593161,-77.2594832131444));
#12612=CARTESIAN_POINT('Ctrl Pts',(-90.7270152190322,98.9178350153006,-77.2137926604239));
#12613=CARTESIAN_POINT('Ctrl Pts',(-91.275429932033,98.6785063270153,-77.2683334201939));
#12614=CARTESIAN_POINT('Ctrl Pts',(-92.3773154492341,98.3741443355135,-77.5617079439358));
#12615=CARTESIAN_POINT('Ctrl Pts',(-92.930279409063,98.3074822374625,-77.8007530507317));
#12616=CARTESIAN_POINT('Ctrl Pts',(-93.4118265169985,98.3074822374625,-78.0787744031257));
#12617=CARTESIAN_POINT('',(-91.4118265169984,105.235685467738,-81.5428760182629));
#12618=CARTESIAN_POINT('Ctrl Pts',(-91.4118265169984,105.235685467738,-81.5428760182628));
#12619=CARTESIAN_POINT('Ctrl Pts',(-90.930279409063,105.235685467738,-81.2648546658689));
#12620=CARTESIAN_POINT('Ctrl Pts',(-90.4235466956197,105.142197830515,-80.9457346914359));
#12621=CARTESIAN_POINT('Ctrl Pts',(-89.5276720287663,104.732917302591,-80.2955389079813));
#12622=CARTESIAN_POINT('Ctrl Pts',(-89.1396330959697,104.416687991642,-79.9632191485941));
#12623=CARTESIAN_POINT('Ctrl Pts',(-88.6191933845126,103.711566927935,-79.3777677293152));
#12624=CARTESIAN_POINT('Ctrl Pts',(-88.4360002798934,103.294551166156,-79.0871156461153));
#12625=CARTESIAN_POINT('Ctrl Pts',(-88.2882811646739,102.403958803926,-78.5394916564604));
#12626=CARTESIAN_POINT('Ctrl Pts',(-88.3237355082,101.931198710495,-78.281198278488));
#12627=CARTESIAN_POINT('Ctrl Pts',(-88.5726881997782,101.068801289506,-77.8499995679938));
#12628=CARTESIAN_POINT('Ctrl Pts',(-88.8022989313345,100.623349028228,-77.6491867686112));
#12629=CARTESIAN_POINT('Ctrl Pts',(-89.1799219644913,100.151183250598,-77.4741046930827));
#12630=CARTESIAN_POINT('Ctrl Pts',(-89.2438824969059,100.076745862652,-77.4478013653234));
#12631=CARTESIAN_POINT('Ctrl Pts',(-89.3105457858516,100.004330985068,-77.4236234448524));
#12632=CARTESIAN_POINT('',(-91.4118265169984,105.235685467738,-81.5428760182629));
#12633=CARTESIAN_POINT('Ctrl Pts',(-81.8660249138711,98.3074822374626,-71.4128027395504));
#12634=CARTESIAN_POINT('Ctrl Pts',(-82.3237270253547,98.3074822374626,-71.6770571768241));
#12635=CARTESIAN_POINT('Ctrl Pts',(-82.7726916110599,98.3818254132719,-72.0253258196487));
#12636=CARTESIAN_POINT('Ctrl Pts',(-83.5294587228727,98.6836749369366,-72.8018086256385));
#12637=CARTESIAN_POINT('Ctrl Pts',(-83.8381825657519,98.9117809702808,-73.2288909422442));
#12638=CARTESIAN_POINT('Ctrl Pts',(-84.2642108337661,99.4513482675956,-74.0139591549906));
#12639=CARTESIAN_POINT('Ctrl Pts',(-84.4147303979509,99.7982897132532,-74.427397105883));
#12640=CARTESIAN_POINT('Ctrl Pts',(-84.5187012892031,100.598975519632,-75.1573598769691));
#12641=CARTESIAN_POINT('Ctrl Pts',(-84.4719272936971,101.053974393027,-75.4725395573331));
#12642=CARTESIAN_POINT('Ctrl Pts',(-84.2144142894456,101.946025606974,-75.9185651643065));
#12643=CARTESIAN_POINT('Ctrl Pts',(-83.9900828414982,102.430163538118,-76.072953886212));
#12644=CARTESIAN_POINT('Ctrl Pts',(-83.3943596113716,103.332957803082,-76.1947311507971));
#12645=CARTESIAN_POINT('Ctrl Pts',(-83.022912997837,103.751330105905,-76.1639500741449));
#12646=CARTESIAN_POINT('Ctrl Pts',(-82.2465265160762,104.425439262707,-75.9857200884568));
#12647=CARTESIAN_POINT('Ctrl Pts',(-81.7851543098186,104.72612267149,-75.8230324929145));
#12648=CARTESIAN_POINT('Ctrl Pts',(-80.8241649502783,105.131719766025,-75.4002729960248));
#12649=CARTESIAN_POINT('Ctrl Pts',(-80.3237270253549,105.235685467738,-75.1411587919613));
#12650=CARTESIAN_POINT('Ctrl Pts',(-79.8660249138712,105.235685467738,-74.8769043546876));
#12651=CARTESIAN_POINT('Origin',(-119.078493020361,109.,-80.7499999999988));
#12652=CARTESIAN_POINT('',(-104.90435628947,98.3074822374622,-84.7139895609318));
#12653=CARTESIAN_POINT('',(-104.90435628947,98.3074822374623,-84.7139895609318));
#12654=CARTESIAN_POINT('',(-99.9488699419194,100.228885141061,-83.7562504402684));
#12655=CARTESIAN_POINT('Ctrl Pts',(-99.9488699419193,100.228885141061,-83.7562504402685));
#12656=CARTESIAN_POINT('Ctrl Pts',(-100.269274778488,99.8589135037763,-83.6332987009061));
#12657=CARTESIAN_POINT('Ctrl Pts',(-100.672060551272,99.5388009858237,-83.5687616798079));
#12658=CARTESIAN_POINT('Ctrl Pts',(-101.656557156406,98.9446450743508,-83.5546921849167));
#12659=CARTESIAN_POINT('Ctrl Pts',(-102.323796076877,98.6892023001508,-83.659021954752));
#12660=CARTESIAN_POINT('Ctrl Pts',(-103.656688844209,98.3714816818226,-84.070990296531));
#12661=CARTESIAN_POINT('Ctrl Pts',(-104.322168303632,98.3074822374624,-84.3778631705889));
#12662=CARTESIAN_POINT('Ctrl Pts',(-104.90435628947,98.3074822374624,-84.7139895609318));
#12663=CARTESIAN_POINT('',(-102.90435628947,105.235685467738,-88.1780911760691));
#12664=CARTESIAN_POINT('Ctrl Pts',(-102.90435628947,105.235685467738,-88.178091176069));
#12665=CARTESIAN_POINT('Ctrl Pts',(-102.322168303632,105.235685467738,-87.8419647857261));
#12666=CARTESIAN_POINT('Ctrl Pts',(-101.701146422792,105.145679342323,-87.4580891267805));
#12667=CARTESIAN_POINT('Ctrl Pts',(-100.583248552382,104.718635790978,-86.6737387001651));
#12668=CARTESIAN_POINT('Ctrl Pts',(-100.087436405043,104.380238803494,-86.2724890494876));
#12669=CARTESIAN_POINT('Ctrl Pts',(-99.4797157079115,103.63823946452,-85.6153691751923));
#12670=CARTESIAN_POINT('Ctrl Pts',(-99.2762414496599,103.243002384244,-85.320427254354));
#12671=CARTESIAN_POINT('Ctrl Pts',(-99.0952115751188,102.385815407921,-84.7678773474479));
#12672=CARTESIAN_POINT('Ctrl Pts',(-99.1179825761209,101.924673720388,-84.5089097354468));
#12673=CARTESIAN_POINT('Ctrl Pts',(-99.3631680629044,101.075326279613,-84.0842360150593));
#12674=CARTESIAN_POINT('Ctrl Pts',(-99.5989917777891,100.640669594177,-83.8953044405758));
#12675=CARTESIAN_POINT('Ctrl Pts',(-99.9319639746297,100.248502859387,-83.7627974003584));
#12676=CARTESIAN_POINT('Ctrl Pts',(-99.940389585881,100.238677412744,-83.7595046811735));
#12677=CARTESIAN_POINT('Ctrl Pts',(-99.9488699419193,100.228885141061,-83.7562504402685));
#12678=CARTESIAN_POINT('',(-102.90435628947,105.235685467738,-88.1780911760691));
#12679=CARTESIAN_POINT('Ctrl Pts',(-93.4118265169985,98.3074822374625,-78.0787744031257));
#12680=CARTESIAN_POINT('Ctrl Pts',(-93.9211136281798,98.3074822374625,-78.372811453861));
#12681=CARTESIAN_POINT('Ctrl Pts',(-94.4293110479316,98.3809411378057,-78.7542137874603));
#12682=CARTESIAN_POINT('Ctrl Pts',(-95.3131003585774,98.6801492903014,-79.6011997737382));
#12683=CARTESIAN_POINT('Ctrl Pts',(-95.68953602647,98.9062732240902,-80.0657700699796));
#12684=CARTESIAN_POINT('Ctrl Pts',(-96.2180755930993,99.439773757549,-80.9039616912801));
#12685=CARTESIAN_POINT('Ctrl Pts',(-96.4211158671793,99.7760817327783,-81.3392544545395));
#12686=CARTESIAN_POINT('Ctrl Pts',(-96.603988459357,100.572512615503,-82.1140272198499));
#12687=CARTESIAN_POINT('Ctrl Pts',(-96.5825452086925,101.034655609006,-82.4517288812605));
#12688=CARTESIAN_POINT('Ctrl Pts',(-96.3138784992858,101.965344390996,-82.9170732722552));
#12689=CARTESIAN_POINT('Ctrl Pts',(-96.0594130029196,102.458977333713,-83.0572595789545));
#12690=CARTESIAN_POINT('Ctrl Pts',(-95.3867915721352,103.359086193817,-83.1307566850585));
#12691=CARTESIAN_POINT('Ctrl Pts',(-94.9692620595266,103.765790736204,-83.0669701806072));
#12692=CARTESIAN_POINT('Ctrl Pts',(-94.0943036219507,104.432320373106,-82.8287936444868));
#12693=CARTESIAN_POINT('Ctrl Pts',(-93.5664254574151,104.730808636538,-82.6265294468561));
#12694=CARTESIAN_POINT('Ctrl Pts',(-92.4801710348681,105.132960205189,-82.130223321151));
#12695=CARTESIAN_POINT('Ctrl Pts',(-91.9211136281798,105.235685467738,-81.8369130689982));
#12696=CARTESIAN_POINT('Ctrl Pts',(-91.4118265169984,105.235685467738,-81.5428760182629));
#12697=CARTESIAN_POINT('Origin',(-119.078493020361,109.,-80.7499999999988));
#12698=CARTESIAN_POINT('',(-106.270002469182,105.235685467738,-90.1212479039226));
#12699=CARTESIAN_POINT('',(-106.270002469182,105.235685467738,-90.1212479039226));
#12700=CARTESIAN_POINT('Ctrl Pts',(-104.90435628947,98.3074822374624,-84.7139895609318));
#12701=CARTESIAN_POINT('Ctrl Pts',(-105.520546937821,98.3074822374624,-85.0697473976293));
#12702=CARTESIAN_POINT('Ctrl Pts',(-106.150726410955,98.3786464989181,-85.5188532090103));
#12703=CARTESIAN_POINT('Ctrl Pts',(-107.289220969567,98.6734920739597,-86.5082604731963));
#12704=CARTESIAN_POINT('Ctrl Pts',(-107.798461931632,98.8969623992174,-87.0475589280851));
#12705=CARTESIAN_POINT('Ctrl Pts',(-108.520316145588,99.4223913020677,-87.9892961628252));
#12706=CARTESIAN_POINT('Ctrl Pts',(-108.815648667087,99.7399146036544,-88.4622960553437));
#12707=CARTESIAN_POINT('Ctrl Pts',(-109.06520359177,100.328003547478,-89.1041494241911));
#12708=CARTESIAN_POINT('Ctrl Pts',(-109.116864532686,100.542611823444,-89.3070609778502));
#12709=CARTESIAN_POINT('Ctrl Pts',(-109.140178467765,101.001678002652,-89.6682684715672));
#12710=CARTESIAN_POINT('Ctrl Pts',(-109.111806983136,101.246175947599,-89.8265150985448));
#12711=CARTESIAN_POINT('Ctrl Pts',(-108.965261598155,101.753824052402,-90.080339150946));
#12712=CARTESIAN_POINT('Ctrl Pts',(-108.849954531701,102.007043208325,-90.1709510744033));
#12713=CARTESIAN_POINT('Ctrl Pts',(-108.552569635501,102.497386688197,-90.2844484102263));
#12714=CARTESIAN_POINT('Ctrl Pts',(-108.370506562727,102.734504647816,-90.3073999743598));
#12715=CARTESIAN_POINT('Ctrl Pts',(-107.75853069038,103.401878694155,-90.2932781005938));
#12716=CARTESIAN_POINT('Ctrl Pts',(-107.260215630608,103.787507531247,-90.1718542774143));
#12717=CARTESIAN_POINT('Ctrl Pts',(-106.197183712277,104.44395286517,-89.8210541610607));
#12718=CARTESIAN_POINT('Ctrl Pts',(-105.538070840598,104.739654064067,-89.5413414682492));
#12719=CARTESIAN_POINT('Ctrl Pts',(-104.200003266355,105.136149694813,-88.8976048069571));
#12720=CARTESIAN_POINT('Ctrl Pts',(-103.520546937821,105.235685467738,-88.5338490127664));
#12721=CARTESIAN_POINT('Ctrl Pts',(-102.90435628947,105.235685467738,-88.178091176069));
#12722=CARTESIAN_POINT('',(-108.270002469182,98.3074822374624,-86.6571462887851));
#12723=CARTESIAN_POINT('',(-108.270002469182,98.3074822374623,-86.6571462887851));
#12724=CARTESIAN_POINT('Ctrl Pts',(-106.270002469182,105.235685467738,-90.1212479039226));
#12725=CARTESIAN_POINT('Ctrl Pts',(-106.398364251285,105.235685467738,-90.1953576133737));
#12726=CARTESIAN_POINT('Ctrl Pts',(-106.527960736738,105.218918283964,-90.2651932010029));
#12727=CARTESIAN_POINT('Ctrl Pts',(-106.847366026658,105.139174343852,-90.425397613589));
#12728=CARTESIAN_POINT('Ctrl Pts',(-107.033287150629,105.059113530962,-90.5082215504996));
#12729=CARTESIAN_POINT('Ctrl Pts',(-107.487244640969,104.791037335221,-90.6836023495469));
#12730=CARTESIAN_POINT('Ctrl Pts',(-107.742055343965,104.569575136487,-90.7553778221103));
#12731=CARTESIAN_POINT('Ctrl Pts',(-108.312044999287,103.952474510198,-90.8506321914898));
#12732=CARTESIAN_POINT('Ctrl Pts',(-108.601687275107,103.516179693072,-90.83222067748));
#12733=CARTESIAN_POINT('Ctrl Pts',(-109.016285784176,102.748005272445,-90.6902990309755));
#12734=CARTESIAN_POINT('Ctrl Pts',(-109.166799177582,102.411600006565,-90.5937735724328));
#12735=CARTESIAN_POINT('Ctrl Pts',(-109.364309285276,101.886060973467,-90.3923049613581));
#12736=CARTESIAN_POINT('Ctrl Pts',(-109.428881856401,101.691891969437,-90.3067091143765));
#12737=CARTESIAN_POINT('Ctrl Pts',(-109.539343060738,101.309363471567,-90.1154913997023));
#12738=CARTESIAN_POINT('Ctrl Pts',(-109.58547134865,101.12019828098,-90.0094768684831));
#12739=CARTESIAN_POINT('Ctrl Pts',(-109.683806016576,100.621556930253,-89.6991065970049));
#12740=CARTESIAN_POINT('Ctrl Pts',(-109.718746169311,100.316400657043,-89.4751827475122));
#12741=CARTESIAN_POINT('Ctrl Pts',(-109.719931149862,99.6457292128168,-88.8981274115455));
#12742=CARTESIAN_POINT('Ctrl Pts',(-109.659507933391,99.2872907854466,-88.5188240602725));
#12743=CARTESIAN_POINT('Ctrl Pts',(-109.407078555524,98.8025861049536,-87.8721136642323));
#12744=CARTESIAN_POINT('Ctrl Pts',(-109.264504916411,98.6353091816041,-87.6059682053067));
#12745=CARTESIAN_POINT('Ctrl Pts',(-108.94540320403,98.4361359224893,-87.1969059803222));
#12746=CARTESIAN_POINT('Ctrl Pts',(-108.799409958408,98.3776732407719,-87.0447641078801));
#12747=CARTESIAN_POINT('Ctrl Pts',(-108.519683286228,98.3196123402596,-86.8155806823361));
#12748=CARTESIAN_POINT('Ctrl Pts',(-108.39839753492,98.3074822374624,-86.7312752145517));
#12749=CARTESIAN_POINT('Ctrl Pts',(-108.270002469182,98.3074822374624,-86.6571462887851));
#12750=CARTESIAN_POINT('Origin',(-119.078493020361,109.,-80.7499999999988));
#12751=CARTESIAN_POINT('',(-85.1260169266464,123.456832294801,-65.7663309411545));
#12752=CARTESIAN_POINT('',(-73.5607164801933,123.456832294801,-59.0891016151359));
#12753=CARTESIAN_POINT('',(-85.1260169266463,123.456832294801,-65.7663309411548));
#12754=CARTESIAN_POINT('',(-83.1162922298706,123.872941359692,-62.2368404208554));
#12755=CARTESIAN_POINT('Ctrl Pts',(-83.1162922298706,123.872941359692,-62.2368404208554));
#12756=CARTESIAN_POINT('Ctrl Pts',(-83.1062743831766,123.829770440363,-62.6116107413721));
#12757=CARTESIAN_POINT('Ctrl Pts',(-83.1509026868771,123.7792071983,-62.9828538443025));
#12758=CARTESIAN_POINT('Ctrl Pts',(-83.3664532434541,123.66173721786,-63.8135927138417));
#12759=CARTESIAN_POINT('Ctrl Pts',(-83.6030554954123,123.587986446344,-64.3071289633042));
#12760=CARTESIAN_POINT('Ctrl Pts',(-84.2623538476765,123.484750532966,-65.1560397594667));
#12761=CARTESIAN_POINT('Ctrl Pts',(-84.6849506657898,123.456832294801,-65.5116812167184));
#12762=CARTESIAN_POINT('Ctrl Pts',(-85.1260169266465,123.456832294801,-65.7663309411545));
#12763=CARTESIAN_POINT('',(-89.1260169266464,123.456832294801,-58.8381277108788));
#12764=CARTESIAN_POINT('Ctrl Pts',(-89.1260169266463,123.456832294801,-58.8381277108789));
#12765=CARTESIAN_POINT('Ctrl Pts',(-88.6849506657896,123.456832294801,-58.5834779864428));
#12766=CARTESIAN_POINT('Ctrl Pts',(-88.165657720114,123.484750532965,-58.395319135024));
#12767=CARTESIAN_POINT('Ctrl Pts',(-87.1008302289584,123.587986446343,-58.2488054113713));
#12768=CARTESIAN_POINT('Ctrl Pts',(-86.5551141732562,123.66173721786,-58.2906699753141));
#12769=CARTESIAN_POINT('Ctrl Pts',(-85.5888213740156,123.798956955934,-58.5578170932871));
#12770=CARTESIAN_POINT('Ctrl Pts',(-85.1044718647574,123.871021105468,-58.7975024013151));
#12771=CARTESIAN_POINT('Ctrl Pts',(-84.2687404142013,123.972199967385,-59.4532843052146));
#12772=CARTESIAN_POINT('Ctrl Pts',(-83.9170521365101,124.,-59.8691926348772));
#12773=CARTESIAN_POINT('Ctrl Pts',(-83.4144629487118,124.,-60.7397026434787));
#12774=CARTESIAN_POINT('Ctrl Pts',(-83.2301199084241,123.972199967385,-61.2522277910038));
#12775=CARTESIAN_POINT('Ctrl Pts',(-83.1333491468145,123.906950854201,-61.9304287037879));
#12776=CARTESIAN_POINT('Ctrl Pts',(-83.120379607442,123.890555509,-62.0839305341979));
#12777=CARTESIAN_POINT('Ctrl Pts',(-83.1162922298706,123.872941359692,-62.2368404208553));
#12778=CARTESIAN_POINT('',(-77.5607164801934,123.456832294801,-52.1608983848601));
#12779=CARTESIAN_POINT('',(-89.1260169266463,123.456832294801,-58.8381277108789));
#12780=CARTESIAN_POINT('',(-75.5607164801928,123.594519519327,-59.6249999999981));
#12781=CARTESIAN_POINT('Ctrl Pts',(-75.5607164801923,123.594519519327,-59.6249999999981));
#12782=CARTESIAN_POINT('Ctrl Pts',(-75.9177670555452,123.636893626714,-59.6249999999981));
#12783=CARTESIAN_POINT('Ctrl Pts',(-76.270167318939,123.685122421852,-59.576007942327));
#12784=CARTESIAN_POINT('Ctrl Pts',(-77.0792037993761,123.798839176147,-59.3592272707466));
#12785=CARTESIAN_POINT('Ctrl Pts',(-77.5695548504124,123.870716769224,-59.1248365924091));
#12786=CARTESIAN_POINT('Ctrl Pts',(-78.4161592503826,123.971970182233,-58.476444301003));
#12787=CARTESIAN_POINT('Ctrl Pts',(-78.7723947994248,124.,-58.0622099735219));
#12788=CARTESIAN_POINT('Ctrl Pts',(-79.2772413912376,124.,-57.1877900264742));
#12789=CARTESIAN_POINT('Ctrl Pts',(-79.4578610674346,123.971970182233,-56.672163827532));
#12790=CARTESIAN_POINT('Ctrl Pts',(-79.5960830634252,123.870716769223,-55.6147867644991));
#12791=CARTESIAN_POINT('Ctrl Pts',(-79.5538958197575,123.798839176147,-55.0729349583605));
#12792=CARTESIAN_POINT('Ctrl Pts',(-79.2949201129009,123.662988149345,-54.1064244624455));
#12793=CARTESIAN_POINT('Ctrl Pts',(-79.0605274269875,123.589960152211,-53.6161302759907));
#12794=CARTESIAN_POINT('Ctrl Pts',(-78.4121993371972,123.486046379795,-52.7696054406997));
#12795=CARTESIAN_POINT('Ctrl Pts',(-77.9980062737959,123.456832294801,-52.4133677649104));
#12796=CARTESIAN_POINT('Ctrl Pts',(-77.5607164801933,123.456832294801,-52.1608983848601));
#12797=CARTESIAN_POINT('Ctrl Pts',(-73.5607164801933,123.456832294801,-59.0891016151359));
#12798=CARTESIAN_POINT('Ctrl Pts',(-73.9980062737958,123.456832294801,-59.3415709951862));
#12799=CARTESIAN_POINT('Ctrl Pts',(-74.5136136825151,123.486046379796,-59.5221538722684));
#12800=CARTESIAN_POINT('Ctrl Pts',(-75.214498480876,123.554932441228,-59.6137729046024));
#12801=CARTESIAN_POINT('Ctrl Pts',(-75.3881510574346,123.57403977147,-59.6249999999981));
#12802=CARTESIAN_POINT('Ctrl Pts',(-75.5607164801923,123.594519519327,-59.6249999999981));
#12803=CARTESIAN_POINT('Origin',(-119.078493020361,109.,-80.7499999999988));
#12804=CARTESIAN_POINT('',(-96.6718185297735,123.456832294801,-72.4323026047302));
#12805=CARTESIAN_POINT('',(-96.6718185297736,123.456832294801,-72.4323026047302));
#12806=CARTESIAN_POINT('',(-94.4177421038261,123.892951352905,-68.5776999378933));
#12807=CARTESIAN_POINT('Ctrl Pts',(-94.4177421038264,123.892951352906,-68.5776999378912));
#12808=CARTESIAN_POINT('Ctrl Pts',(-94.3950722235507,123.847611592354,-69.0004788607279));
#12809=CARTESIAN_POINT('Ctrl Pts',(-94.4446100038828,123.791696326041,-69.4229013343407));
#12810=CARTESIAN_POINT('Ctrl Pts',(-94.6962798517419,123.665476993059,-70.3388246478844));
#12811=CARTESIAN_POINT('Ctrl Pts',(-94.9708319480395,123.588576370395,-70.867709374078));
#12812=CARTESIAN_POINT('Ctrl Pts',(-95.7182701307845,123.483657833973,-71.7750046897054));
#12813=CARTESIAN_POINT('Ctrl Pts',(-96.1902714218383,123.456832294801,-72.154281252336));
#12814=CARTESIAN_POINT('Ctrl Pts',(-96.6718185297737,123.456832294801,-72.43230260473));
#12815=CARTESIAN_POINT('',(-100.671818529773,123.456832294801,-65.5040993744542));
#12816=CARTESIAN_POINT('Ctrl Pts',(-100.671818529773,123.456832294801,-65.5040993744543));
#12817=CARTESIAN_POINT('Ctrl Pts',(-100.198890562852,123.456832294801,-65.2310542854448));
#12818=CARTESIAN_POINT('Ctrl Pts',(-99.6449352638787,123.482663841571,-65.0141879033647));
#12819=CARTESIAN_POINT('Ctrl Pts',(-98.5058533293481,123.584301615867,-64.8160574918001));
#12820=CARTESIAN_POINT('Ctrl Pts',(-97.9204236427471,123.659016564532,-64.8359793331119));
#12821=CARTESIAN_POINT('Ctrl Pts',(-96.9056954794152,123.797787553474,-65.0846768377439));
#12822=CARTESIAN_POINT('Ctrl Pts',(-96.4098673945079,123.869713255231,-65.3135356756117));
#12823=CARTESIAN_POINT('Ctrl Pts',(-95.5559638106463,123.971567821815,-65.9593477666097));
#12824=CARTESIAN_POINT('Ctrl Pts',(-95.1973252908835,124.,-66.3757915444938));
#12825=CARTESIAN_POINT('Ctrl Pts',(-94.6944496907949,124.,-67.2467976337339));
#12826=CARTESIAN_POINT('Ctrl Pts',(-94.5146381715445,123.972692167848,-67.755124974498));
#12827=CARTESIAN_POINT('Ctrl Pts',(-94.4324796442889,123.913947930132,-68.376407921987));
#12828=CARTESIAN_POINT('Ctrl Pts',(-94.4231381300388,123.903743405331,-68.4770674633497));
#12829=CARTESIAN_POINT('Ctrl Pts',(-94.4177421038264,123.892951352906,-68.5776999378912));
#12830=CARTESIAN_POINT('',(-100.671818529773,123.456832294801,-65.5040993744543));
#12831=CARTESIAN_POINT('Ctrl Pts',(-85.1260169266465,123.456832294801,-65.7663309411545));
#12832=CARTESIAN_POINT('Ctrl Pts',(-85.5837190381301,123.456832294801,-66.0305853784282));
#12833=CARTESIAN_POINT('Ctrl Pts',(-86.122720562641,123.486454820705,-66.2229054686833));
#12834=CARTESIAN_POINT('Ctrl Pts',(-87.2307450620227,123.590202391576,-66.3909926328699));
#12835=CARTESIAN_POINT('Ctrl Pts',(-87.7998683754043,123.662779767014,-66.3670498363015));
#12836=CARTESIAN_POINT('Ctrl Pts',(-88.8096922981326,123.797321626501,-66.140954313845));
#12837=CARTESIAN_POINT('Ctrl Pts',(-89.3225329048017,123.868752483667,-65.9268338105032));
#12838=CARTESIAN_POINT('Ctrl Pts',(-90.208346563904,123.970860942253,-65.3026051841426));
#12839=CARTESIAN_POINT('Ctrl Pts',(-90.5808483157038,124.,-64.8915779677916));
#12840=CARTESIAN_POINT('Ctrl Pts',(-91.095874324207,124.,-63.9995267538447));
#12841=CARTESIAN_POINT('Ctrl Pts',(-91.2655834593138,123.970860942253,-63.4714171656563));
#12842=CARTESIAN_POINT('Ctrl Pts',(-91.3632744779603,123.868752483666,-62.3921657206742));
#12843=CARTESIAN_POINT('Ctrl Pts',(-91.2922879699909,123.797321626501,-61.8409724755356));
#12844=CARTESIAN_POINT('Ctrl Pts',(-90.9831804747559,123.662779767014,-60.8533915438754));
#12845=CARTESIAN_POINT('Ctrl Pts',(-90.7193538881309,123.590202391575,-60.3485448983168));
#12846=CARTESIAN_POINT('Ctrl Pts',(-90.0197738842044,123.486454820704,-59.47301111593));
#12847=CARTESIAN_POINT('Ctrl Pts',(-89.5837190381299,123.456832294801,-59.1023821481526));
#12848=CARTESIAN_POINT('Ctrl Pts',(-89.1260169266463,123.456832294801,-58.8381277108788));
#12849=CARTESIAN_POINT('Origin',(-119.078493020361,109.,-80.7499999999988));
#12850=CARTESIAN_POINT('',(-108.164348302245,123.456832294801,-79.0675177625366));
#12851=CARTESIAN_POINT('',(-108.164348302245,123.456832294801,-79.0675177625365));
#12852=CARTESIAN_POINT('',(-105.277091391218,123.923615035047,-74.5275001761057));
#12853=CARTESIAN_POINT('Ctrl Pts',(-105.277091391218,123.923615035047,-74.5275001761056));
#12854=CARTESIAN_POINT('Ctrl Pts',(-105.275365738248,123.921622422635,-74.5492158639596));
#12855=CARTESIAN_POINT('Ctrl Pts',(-105.273837242761,123.919598892701,-74.5709499461767));
#12856=CARTESIAN_POINT('Ctrl Pts',(-105.238853605271,123.865658954398,-75.1423248070353));
#12857=CARTESIAN_POINT('Ctrl Pts',(-105.33860750079,123.794453706366,-75.701175262549));
#12858=CARTESIAN_POINT('Ctrl Pts',(-105.746737061739,123.654133883405,-76.7806745481755));
#12859=CARTESIAN_POINT('Ctrl Pts',(-106.120272716169,123.5787523934,-77.3509626000236));
#12860=CARTESIAN_POINT('Ctrl Pts',(-107.054281271328,123.479989785222,-78.3346823431572));
#12861=CARTESIAN_POINT('Ctrl Pts',(-107.613395871184,123.456832294801,-78.7494252281526));
#12862=CARTESIAN_POINT('Ctrl Pts',(-108.164348302246,123.456832294801,-79.0675177625365));
#12863=CARTESIAN_POINT('',(-112.164348302245,123.456832294801,-72.1393145322606));
#12864=CARTESIAN_POINT('Ctrl Pts',(-112.164348302245,123.456832294801,-72.1393145322606));
#12865=CARTESIAN_POINT('Ctrl Pts',(-111.613395871184,123.456832294801,-71.8212219978767));
#12866=CARTESIAN_POINT('Ctrl Pts',(-110.974660696811,123.479989785221,-71.5443859932717));
#12867=CARTESIAN_POINT('Ctrl Pts',(-109.655730131473,123.578752393399,-71.2273707287195));
#12868=CARTESIAN_POINT('Ctrl Pts',(-108.975078363883,123.654133883405,-71.1890233886878));
#12869=CARTESIAN_POINT('Ctrl Pts',(-107.836139778689,123.794453706366,-71.3753224636836));
#12870=CARTESIAN_POINT('Ctrl Pts',(-107.302284139538,123.865658954397,-71.5683582837951));
#12871=CARTESIAN_POINT('Ctrl Pts',(-106.383953947217,123.96943271423,-72.1762726463728));
#12872=CARTESIAN_POINT('Ctrl Pts',(-105.998960269092,124.,-72.5907067654734));
#12873=CARTESIAN_POINT('Ctrl Pts',(-105.482985495051,124.,-73.4844012895352));
#12874=CARTESIAN_POINT('Ctrl Pts',(-105.318978111356,123.971981653342,-74.0003959692113));
#12875=CARTESIAN_POINT('Ctrl Pts',(-105.277091391218,123.923615035047,-74.5275001761056));
#12876=CARTESIAN_POINT('',(-112.164348302245,123.456832294801,-72.1393145322605));
#12877=CARTESIAN_POINT('Ctrl Pts',(-96.6718185297737,123.456832294801,-72.43230260473));
#12878=CARTESIAN_POINT('Ctrl Pts',(-97.2080109095617,123.456832294801,-72.741873419538));
#12879=CARTESIAN_POINT('Ctrl Pts',(-97.8378331599511,123.489300624785,-72.9756291788421));
#12880=CARTESIAN_POINT('Ctrl Pts',(-99.1346770015159,123.601479985038,-73.210267194341));
#12881=CARTESIAN_POINT('Ctrl Pts',(-99.801733680399,123.679673134231,-73.2116784585455));
#12882=CARTESIAN_POINT('Ctrl Pts',(-100.899904621245,123.812998388381,-73.0077930813484));
#12883=CARTESIAN_POINT('Ctrl Pts',(-101.417162434113,123.877803175384,-72.8258148556167));
#12884=CARTESIAN_POINT('Ctrl Pts',(-102.313026843884,123.972069837582,-72.2590940486296));
#12885=CARTESIAN_POINT('Ctrl Pts',(-102.69054002654,124.,-71.8723715243807));
#12886=CARTESIAN_POINT('Ctrl Pts',(-103.196264738206,124.,-70.9964306291323));
#12887=CARTESIAN_POINT('Ctrl Pts',(-103.342419677093,123.972069837582,-70.4761333605637));
#12888=CARTESIAN_POINT('Ctrl Pts',(-103.385282087912,123.877803175384,-69.4169316198625));
#12889=CARTESIAN_POINT('Ctrl Pts',(-103.284250947897,123.812998388381,-68.8779841007473));
#12890=CARTESIAN_POINT('Ctrl Pts',(-102.911735393587,123.67967313423,-67.8249974796778));
#12891=CARTESIAN_POINT('Ctrl Pts',(-102.576984863492,123.601479985038,-67.2480150821033));
#12892=CARTESIAN_POINT('Ctrl Pts',(-101.725360460594,123.489300624784,-66.2422343783163));
#12893=CARTESIAN_POINT('Ctrl Pts',(-101.208010909561,123.456832294801,-65.8136701892623));
#12894=CARTESIAN_POINT('Ctrl Pts',(-100.671818529773,123.456832294801,-65.5040993744543));
#12895=CARTESIAN_POINT('Origin',(-119.078493020361,109.,-80.7499999999988));
#12896=CARTESIAN_POINT('',(-115.529994481957,123.456832294801,-74.0824712601142));
#12897=CARTESIAN_POINT('',(-115.529994481957,123.456832294801,-74.082471260114));
#12898=CARTESIAN_POINT('Ctrl Pts',(-108.164348302246,123.456832294801,-79.0675177625365));
#12899=CARTESIAN_POINT('Ctrl Pts',(-108.844463055017,123.456832294801,-79.4601821981288));
#12900=CARTESIAN_POINT('Ctrl Pts',(-109.637912977074,123.491441900927,-79.7804741154724));
#12901=CARTESIAN_POINT('Ctrl Pts',(-111.275183810088,123.611693066724,-80.170706138189));
#12902=CARTESIAN_POINT('Ctrl Pts',(-112.118571906507,123.696010228407,-80.2428658921871));
#12903=CARTESIAN_POINT('Ctrl Pts',(-113.398550856209,123.828649318389,-80.1045968599479));
#12904=CARTESIAN_POINT('Ctrl Pts',(-113.937605814753,123.885984825864,-79.974373351834));
#12905=CARTESIAN_POINT('Ctrl Pts',(-114.643393821985,123.950735654834,-79.6153146748024));
#12906=CARTESIAN_POINT('Ctrl Pts',(-114.862132214305,123.968740024147,-79.4686771786292));
#12907=CARTESIAN_POINT('Ctrl Pts',(-115.243722739859,123.993392806363,-79.1229603686417));
#12908=CARTESIAN_POINT('Ctrl Pts',(-115.406496999395,124.,-78.9237921724865));
#12909=CARTESIAN_POINT('Ctrl Pts',(-115.660952638663,124.,-78.4830620770019));
#12910=CARTESIAN_POINT('Ctrl Pts',(-115.752050226392,123.993392806363,-78.2425113350836));
#12911=CARTESIAN_POINT('Ctrl Pts',(-115.860654503579,123.968740024147,-77.7391858411162));
#12912=CARTESIAN_POINT('Ctrl Pts',(-115.878277104252,123.950735654834,-77.4764340884979));
#12913=CARTESIAN_POINT('Ctrl Pts',(-115.836337036395,123.885984825864,-76.6856744060329));
#12914=CARTESIAN_POINT('Ctrl Pts',(-115.679586423319,123.828649318388,-76.1537273638406));
#12915=CARTESIAN_POINT('Ctrl Pts',(-115.159341442944,123.696010228406,-74.9760985609694));
#12916=CARTESIAN_POINT('Ctrl Pts',(-114.675155214641,123.611693066724,-74.2817829212208));
#12917=CARTESIAN_POINT('Ctrl Pts',(-113.518568953091,123.491441900926,-73.0589807983134));
#12918=CARTESIAN_POINT('Ctrl Pts',(-112.844463055016,123.456832294801,-72.531978967853));
#12919=CARTESIAN_POINT('Ctrl Pts',(-112.164348302245,123.456832294801,-72.1393145322606));
#12920=CARTESIAN_POINT('',(-111.529994481957,123.456832294801,-81.0106744903897));
#12921=CARTESIAN_POINT('',(-111.529994481957,123.456832294801,-81.0106744903897));
#12922=CARTESIAN_POINT('Ctrl Pts',(-115.529994481957,123.456832294801,-74.0824712601142));
#12923=CARTESIAN_POINT('Ctrl Pts',(-115.65835626406,123.456832294801,-74.1565809695654));
#12924=CARTESIAN_POINT('Ctrl Pts',(-115.77745320865,123.461475653088,-74.2446022954246));
#12925=CARTESIAN_POINT('Ctrl Pts',(-116.046607194207,123.483194384997,-74.4918445203156));
#12926=CARTESIAN_POINT('Ctrl Pts',(-116.181936272838,123.504836535895,-74.6622964502142));
#12927=CARTESIAN_POINT('Ctrl Pts',(-116.463492476953,123.573840873615,-75.1362850362945));
#12928=CARTESIAN_POINT('Ctrl Pts',(-116.573472758241,123.62806730643,-75.4589141577373));
#12929=CARTESIAN_POINT('Ctrl Pts',(-116.724373411066,123.761245635907,-76.2800519723337));
#12930=CARTESIAN_POINT('Ctrl Pts',(-116.704520006728,123.840165624527,-76.7977027010819));
#12931=CARTESIAN_POINT('Ctrl Pts',(-116.53883398008,123.93828517935,-77.6608633532843));
#12932=CARTESIAN_POINT('Ctrl Pts',(-116.424541973442,123.968919507233,-78.0229943017362));
#12933=CARTESIAN_POINT('Ctrl Pts',(-116.189563012637,123.995063180093,-78.5706187310189));
#12934=CARTESIAN_POINT('Ctrl Pts',(-116.090247091074,123.99999005338,-78.7688860801498));
#12935=CARTESIAN_POINT('Ctrl Pts',(-115.86944609645,124.000009911765,-79.1514313247033));
#12936=CARTESIAN_POINT('Ctrl Pts',(-115.74750688821,123.995107474062,-79.3365182359193));
#12937=CARTESIAN_POINT('Ctrl Pts',(-115.391456612351,123.969070285569,-79.8131657732718));
#12938=CARTESIAN_POINT('Ctrl Pts',(-115.135714858818,123.938576005114,-80.0927177542768));
#12939=CARTESIAN_POINT('Ctrl Pts',(-114.471237782264,123.840607113622,-80.6686229218872));
#12940=CARTESIAN_POINT('Ctrl Pts',(-114.031900126614,123.761512834073,-80.9456186309926));
#12941=CARTESIAN_POINT('Ctrl Pts',(-113.24419775823,123.628137504237,-81.2260282504464));
#12942=CARTESIAN_POINT('Ctrl Pts',(-112.909789654842,123.573903068408,-81.292149830288));
#12943=CARTESIAN_POINT('Ctrl Pts',(-112.358412824606,123.504868123884,-81.2853999107625));
#12944=CARTESIAN_POINT('Ctrl Pts',(-112.143032917437,123.483209990156,-81.2534392614886));
#12945=CARTESIAN_POINT('Ctrl Pts',(-111.794203638433,123.461478073366,-81.1439450618975));
#12946=CARTESIAN_POINT('Ctrl Pts',(-111.658389547695,123.456832294801,-81.0848034161563));
#12947=CARTESIAN_POINT('Ctrl Pts',(-111.529994481957,123.456832294801,-81.0106744903897));
#12948=CARTESIAN_POINT('Origin',(-119.078493020361,109.,-80.7499999999988));
#12949=CARTESIAN_POINT('',(-126.564449609913,108.0824948189,-67.7839428436388));
#12950=CARTESIAN_POINT('',(-122.424179917669,122.42480974691,-74.9551003076436));
#12951=CARTESIAN_POINT('Origin',(-119.078493020361,109.,-80.7499999999988));
#12952=CARTESIAN_POINT('',(-77.2010015942,108.0824948189,-39.2839428436393));
#12953=CARTESIAN_POINT('',(-126.564449609913,108.0824948189,-67.7839428436388));
#12954=CARTESIAN_POINT('',(-73.0607319019557,122.42480974691,-46.4551003076441));
#12955=CARTESIAN_POINT('Origin',(-69.7150450046476,109.,-52.2499999999992));
#12956=CARTESIAN_POINT('',(-122.424179917669,122.42480974691,-74.9551003076436));
#12957=CARTESIAN_POINT('Origin',(-69.7150450046476,109.,-52.2499999999992));
#12958=CARTESIAN_POINT('',(-73.7335498795933,101.937180526609,-39.2897453861299));
#12959=CARTESIAN_POINT('',(-70.2694482644555,101.937180526609,-37.2897453861299));
#12960=CARTESIAN_POINT('',(-73.7335498795933,101.937180526609,-39.2897453861299));
#12961=CARTESIAN_POINT('',(-67.366968793295,123.991664350565,-50.3169872981059));
#12962=CARTESIAN_POINT('Origin',(-67.1169687932943,109.,-50.7499999999993));
#12963=CARTESIAN_POINT('',(-63.9028671781572,123.991664350565,-48.3169872981059));
#12964=CARTESIAN_POINT('',(-67.366968793295,123.991664350565,-50.3169872981059));
#12965=CARTESIAN_POINT('Origin',(-63.6528671781565,109.,-48.7499999999993));
#12966=CARTESIAN_POINT('Origin',(-69.7150450046476,109.,-52.2499999999992));
#12967=CARTESIAN_POINT('',(-78.2150450046475,109.,-37.5275681356637));
#12968=CARTESIAN_POINT('Origin',(-69.7150450046476,109.,-52.2499999999992));
#12969=CARTESIAN_POINT('',(-76.9580463854329,108.363035329266,-39.7047536091873));
#12970=CARTESIAN_POINT('',(-76.9580463854329,108.363035329266,-39.7047536091873));
#12971=CARTESIAN_POINT('',(-73.6123594881249,96.7732359445554,-45.4996533015424));
#12972=CARTESIAN_POINT('Origin',(-69.7150450046476,109.,-52.2499999999992));
#12973=CARTESIAN_POINT('',(-73.6123594881249,96.7732359445554,-45.4996533015424));
#12974=CARTESIAN_POINT('',(-65.8177305211704,96.7732359445554,-59.0003466984559));
#12975=CARTESIAN_POINT('',(-65.8177305211704,96.7732359445554,-59.0003466984559));
#12976=CARTESIAN_POINT('',(-62.4720436238624,108.363035329266,-64.7952463908111));
#12977=CARTESIAN_POINT('Origin',(-69.7150450046476,109.,-52.2499999999992));
#12978=CARTESIAN_POINT('',(-62.4720436238624,108.363035329266,-64.7952463908111));
#12979=CARTESIAN_POINT('',(-66.3693581073396,121.863728726179,-58.0448996923544));
#12980=CARTESIAN_POINT('',(-66.3693581073396,121.863728726179,-58.0448996923544));
#12981=CARTESIAN_POINT('',(-73.0607319019557,121.863728726179,-46.4551003076441));
#12982=CARTESIAN_POINT('Origin',(-69.7150450046476,109.,-52.2499999999992));
#12983=CARTESIAN_POINT('',(-73.0607319019557,121.863728726179,-46.4551003076441));
#12984=CARTESIAN_POINT('Origin',(-63.6528671781565,109.,-48.7499999999993));
#12985=CARTESIAN_POINT('',(-72.1528671781564,109.,-34.0275681356638));
#12986=CARTESIAN_POINT('Origin',(-63.6528671781565,109.,-48.7499999999993));
#12987=CARTESIAN_POINT('',(-56.6032733899647,101.437180526611,-60.9602546138697));
#12988=CARTESIAN_POINT('',(-56.6032733899647,101.437180526611,-60.9602546138697));
#12989=CARTESIAN_POINT('',(-56.8532733899647,100.571155122826,-60.5272419119775));
#12990=CARTESIAN_POINT('',(-56.8532733899647,100.571155122826,-60.5272419119775));
#12991=CARTESIAN_POINT('',(-57.2862860918569,101.071155122826,-59.7772419119775));
#12992=CARTESIAN_POINT('',(-70.4524609663477,100.571155122824,-36.9727580880222));
#12993=CARTESIAN_POINT('',(-70.4524609663477,100.571155122824,-36.9727580880222));
#12994=CARTESIAN_POINT('',(-70.7024609663477,101.437180526609,-36.5397453861299));
#12995=CARTESIAN_POINT('',(-70.7024609663477,101.437180526609,-36.53974538613));
#12996=CARTESIAN_POINT('',(-70.2694482644555,101.937180526609,-37.2897453861299));
#12997=CARTESIAN_POINT('',(-63.9028671781572,124.991664350565,-48.3169872981059));
#12998=CARTESIAN_POINT('',(-63.9028671781572,124.991664350565,-48.3169872981059));
#12999=CARTESIAN_POINT('',(-63.4028671781572,124.991664350565,-49.1830127018903));
#13000=CARTESIAN_POINT('',(-63.4028671781572,124.991664350565,-49.1830127018903));
#13001=CARTESIAN_POINT('',(-63.4028671781572,123.991664350565,-49.1830127018903));
#13002=CARTESIAN_POINT('Origin',(-69.7150450046476,109.,-52.2499999999992));
#13003=CARTESIAN_POINT('',(-78.2150450046475,109.,-37.5275681356637));
#13004=CARTESIAN_POINT('Origin',(-67.1169687932943,109.,-50.7499999999993));
#13005=CARTESIAN_POINT('',(-60.3173750051025,100.571155122826,-62.5272419119774));
#13006=CARTESIAN_POINT('',(-60.7503877069946,101.071155122826,-61.7772419119775));
#13007=CARTESIAN_POINT('',(-60.0673750051025,101.437180526611,-62.9602546138697));
#13008=CARTESIAN_POINT('',(-60.3173750051025,100.571155122826,-62.5272419119774));
#13009=CARTESIAN_POINT('',(-60.0673750051025,101.437180526611,-62.9602546138697));
#13010=CARTESIAN_POINT('',(-66.866968793295,124.991664350565,-51.1830127018903));
#13011=CARTESIAN_POINT('',(-66.866968793295,123.991664350565,-51.1830127018903));
#13012=CARTESIAN_POINT('',(-67.366968793295,124.991664350565,-50.3169872981059));
#13013=CARTESIAN_POINT('',(-66.866968793295,124.991664350565,-51.1830127018903));
#13014=CARTESIAN_POINT('',(-67.366968793295,124.991664350565,-50.3169872981059));
#13015=CARTESIAN_POINT('',(-74.1665625814855,101.437180526609,-38.5397453861299));
#13016=CARTESIAN_POINT('',(-73.7335498795933,101.937180526609,-39.2897453861299));
#13017=CARTESIAN_POINT('',(-73.9165625814855,100.571155122824,-38.9727580880221));
#13018=CARTESIAN_POINT('',(-74.1665625814855,101.437180526609,-38.5397453861299));
#13019=CARTESIAN_POINT('',(-73.9165625814855,100.571155122824,-38.9727580880221));
#13020=CARTESIAN_POINT('',(-73.616968793294,109.,-39.4916697508017));
#13021=CARTESIAN_POINT('Origin',(-67.116968793295,109.,-50.7499999999981));
#13022=CARTESIAN_POINT('Origin',(-119.078493020361,109.,-80.7499999999988));
#13023=CARTESIAN_POINT('',(-122.975807503838,96.7732359445554,-73.9996533015419));
#13024=CARTESIAN_POINT('',(-122.975807503838,96.7732359445554,-73.9996533015419));
#13025=CARTESIAN_POINT('',(-126.321494401146,108.363035329266,-68.2047536091869));
#13026=CARTESIAN_POINT('Origin',(-119.078493020361,109.,-80.7499999999988));
#13027=CARTESIAN_POINT('',(-126.564449609913,108.0824948189,-67.7839428436388));
#13028=CARTESIAN_POINT('',(-122.424179917669,121.863728726179,-74.9551003076436));
#13029=CARTESIAN_POINT('',(-122.424179917669,121.863728726179,-74.9551003076436));
#13030=CARTESIAN_POINT('',(-115.732806123053,121.863728726179,-86.5448996923539));
#13031=CARTESIAN_POINT('Origin',(-119.078493020361,109.,-80.7499999999988));
#13032=CARTESIAN_POINT('',(-115.732806123053,122.42480974691,-86.5448996923539));
#13033=CARTESIAN_POINT('',(-111.835491639576,108.363035329266,-93.2952463908107));
#13034=CARTESIAN_POINT('',(-111.835491639576,108.363035329266,-93.2952463908107));
#13035=CARTESIAN_POINT('',(-115.181178536884,96.7732359445553,-87.5003466984555));
#13036=CARTESIAN_POINT('Origin',(-119.078493020361,109.,-80.7499999999988));
#13037=CARTESIAN_POINT('',(-114.938223328117,96.49269543419,-87.9211574640035));
#13038=CARTESIAN_POINT('Origin',(-75.5607164801933,129.,-55.624999999998));
#13039=CARTESIAN_POINT('',(-75.5607164801933,129.,-59.6249999999981));
#13040=CARTESIAN_POINT('Origin',(-75.5607164801933,129.,-55.624999999998));
#13041=CARTESIAN_POINT('',(-75.5607164801933,129.,-59.1249999999981));
#13042=CARTESIAN_POINT('Origin',(-75.5607164801933,129.,-55.624999999998));
#13043=CARTESIAN_POINT('Origin',(-75.5607164801933,-5.00102499999999,-55.624999999998));
#13044=CARTESIAN_POINT('',(-75.5607164801933,-5.00102499999999,-59.6249999999981));
#13045=CARTESIAN_POINT('',(-77.5607164801934,122.937359864766,-52.1608983848606));
#13046=CARTESIAN_POINT('',(-77.5607164801934,122.937359864766,-52.1608983848601));
#13047=CARTESIAN_POINT('',(-73.5607164801933,122.937359864767,-59.0891016151359));
#13048=CARTESIAN_POINT('Ctrl Pts',(-77.5607164801933,122.937359864766,-52.1608983848601));
#13049=CARTESIAN_POINT('Ctrl Pts',(-77.1232537523542,122.937359864766,-51.9083291611818));
#13050=CARTESIAN_POINT('Ctrl Pts',(-76.60754249421,122.967689419789,-51.7277743724565));
#13051=CARTESIAN_POINT('Ctrl Pts',(-75.5502948880754,123.075440885261,-51.5896430799529));
#13052=CARTESIAN_POINT('Ctrl Pts',(-75.008612000326,123.151115999848,-51.6318312278756));
#13053=CARTESIAN_POINT('Ctrl Pts',(-74.0423701006026,123.291794528869,-51.8907349645996));
#13054=CARTESIAN_POINT('Ctrl Pts',(-73.5520995881099,123.366192507349,-52.1250380084307));
#13055=CARTESIAN_POINT('Ctrl Pts',(-72.7054703736856,123.47098799846,-52.7733608760245));
#13056=CARTESIAN_POINT('Ctrl Pts',(-72.3491310307417,123.5,-53.1876291712969));
#13057=CARTESIAN_POINT('Ctrl Pts',(-71.8440986993692,123.5,-54.0623708286991));
#13058=CARTESIAN_POINT('Ctrl Pts',(-71.6635015031528,123.47098799846,-54.5781038996925));
#13059=CARTESIAN_POINT('Ctrl Pts',(-71.5253520371743,123.366192507349,-55.635467740767));
#13060=CARTESIAN_POINT('Ctrl Pts',(-71.5675749052789,123.29179452887,-56.1772059812275));
#13061=CARTESIAN_POINT('Ctrl Pts',(-71.826478642003,123.151115999849,-57.143447880951));
#13062=CARTESIAN_POINT('Ctrl Pts',(-72.060784078038,123.075440885262,-57.6336530964987));
#13063=CARTESIAN_POINT('Ctrl Pts',(-72.709033089471,122.96768941979,-58.4801907352497));
#13064=CARTESIAN_POINT('Ctrl Pts',(-73.1232537523542,122.937359864767,-58.8365323914576));
#13065=CARTESIAN_POINT('Ctrl Pts',(-73.5607164801933,122.937359864767,-59.0891016151359));
#13066=CARTESIAN_POINT('',(-73.5607164801933,122.937359864767,-59.0891016151359));
#13067=CARTESIAN_POINT('Origin',(-88.2037045535141,128.101020514434,-62.924432567491));
#13068=CARTESIAN_POINT('',(-84.3072367627289,129.005199011952,-62.924432567491));
#13069=CARTESIAN_POINT('Origin',(-88.2037045535141,128.101020514434,-62.924432567491));
#13070=CARTESIAN_POINT('',(-84.7942952365771,128.892176699762,-62.9244325674911));
#13071=CARTESIAN_POINT('Origin',(-88.2037045535141,128.101020514434,-62.9244325674911));
#13072=CARTESIAN_POINT('Origin',(-39.9537393796627,-79.8274313593171,-35.0673021859779));
#13073=CARTESIAN_POINT('',(-36.0572715888775,-78.9232528617992,-35.0673021859779));
#13074=CARTESIAN_POINT('Origin',(-100.711351574804,127.535898384862,-70.1457259421618));
#13075=CARTESIAN_POINT('',(-97.1336428108046,129.324752766862,-70.1457259421618));
#13076=CARTESIAN_POINT('Origin',(-100.711351574804,127.535898384862,-70.1457259421618));
#13077=CARTESIAN_POINT('',(-97.5808564063047,129.101145969112,-70.1457259421618));
#13078=CARTESIAN_POINT('Origin',(-100.711351574804,127.535898384862,-70.1457259421618));
#13079=CARTESIAN_POINT('Origin',(24.6400845185815,-123.166973801907,2.2259594296606));
#13080=CARTESIAN_POINT('',(28.2177932825812,-121.378119419907,2.2259594296606));
#13081=CARTESIAN_POINT('Origin',(-113.529994481957,127.343145750508,-77.5465728752519));
#13082=CARTESIAN_POINT('',(-110.506278697883,129.96176043334,-77.5465728752519));
#13083=CARTESIAN_POINT('Origin',(-113.529994481957,127.343145750508,-77.5465728752519));
#13084=CARTESIAN_POINT('',(-110.884243170892,129.634433597986,-77.5465728752519));
#13085=CARTESIAN_POINT('Origin',(-113.529994481957,127.343145750508,-77.5465728752519));
#13086=CARTESIAN_POINT('Origin',(101.486213576105,-120.9361854544,46.5930927272026));
#13087=CARTESIAN_POINT('',(104.509929360179,-118.317570771568,46.5930927272026));
#13088=CARTESIAN_POINT('Origin',(-75.5607164801933,126.,-55.624999999998));
#13089=CARTESIAN_POINT('',(-75.5607164801933,126.,-59.1249999999981));
#13090=CARTESIAN_POINT('Origin',(-75.5607164801933,126.,-55.624999999998));
#13091=CARTESIAN_POINT('',(-75.5607164801933,126.,-58.4249999999981));
#13092=CARTESIAN_POINT('Origin',(-75.5607164801933,126.,-55.624999999998));
#13093=CARTESIAN_POINT('Origin',(-75.5607164801933,126.,-55.624999999998));
#13094=CARTESIAN_POINT('',(-75.5607164801933,126.,-59.1249999999981));
#13095=CARTESIAN_POINT('Origin',(-87.531272949388,125.203243035567,-62.5362039998373));
#13096=CARTESIAN_POINT('',(-84.121863632451,125.994399220895,-62.5362039998373));
#13097=CARTESIAN_POINT('Origin',(-87.531272949388,125.203243035567,-62.5362039998373));
#13098=CARTESIAN_POINT('',(-84.8037454958384,125.836167983829,-62.5362039998373));
#13099=CARTESIAN_POINT('Origin',(-87.531272949388,125.203243035567,-62.5362039998373));
#13100=CARTESIAN_POINT('Origin',(-87.531272949388,125.203243035567,-62.5362039998373));
#13101=CARTESIAN_POINT('',(-84.121863632451,125.994399220895,-62.5362039998373));
#13102=CARTESIAN_POINT('Origin',(-99.4123134691276,124.937822173509,-69.3957259421618));
#13103=CARTESIAN_POINT('',(-96.281818300628,126.503069757759,-69.3957259421618));
#13104=CARTESIAN_POINT('Origin',(-99.4123134691276,124.937822173509,-69.3957259421618));
#13105=CARTESIAN_POINT('',(-96.907917334328,126.190020240909,-69.3957259421618));
#13106=CARTESIAN_POINT('Origin',(-99.4123134691276,124.937822173509,-69.3957259421618));
#13107=CARTESIAN_POINT('Origin',(-99.4123134691276,124.937822173509,-69.3957259421618));
#13108=CARTESIAN_POINT('',(-96.281818300628,126.503069757759,-69.3957259421618));
#13109=CARTESIAN_POINT('Origin',(-147.457758061401,109.,-97.1347763108453));
#13110=CARTESIAN_POINT('',(-122.114391405223,109.,-67.4916697508013));
#13111=CARTESIAN_POINT('Origin',(-115.614391405224,109.,-78.7499999999976));
#13112=CARTESIAN_POINT('',(-153.9577580614,109.,-85.8764460616489));
#13113=CARTESIAN_POINT('',(-117.386134507203,101.605059126311,-67.4270749801284));
#13114=CARTESIAN_POINT('',(-111.565481622863,103.438089404292,-62.8444992851723));
#13115=CARTESIAN_POINT('Ctrl Pts',(-117.386134507204,101.60505912631,-67.4270749801283));
#13116=CARTESIAN_POINT('Ctrl Pts',(-117.384843998764,101.603815224188,-67.4273233385933));
#13117=CARTESIAN_POINT('Ctrl Pts',(-117.383552105126,101.602572260028,-67.4275705183945));
#13118=CARTESIAN_POINT('Ctrl Pts',(-117.105783250958,101.335811456963,-67.4804062339256));
#13119=CARTESIAN_POINT('Ctrl Pts',(-116.763727423833,101.113949509274,-67.4772489203251));
#13120=CARTESIAN_POINT('Ctrl Pts',(-115.970697123411,100.70633252813,-67.3909870285613));
#13121=CARTESIAN_POINT('Ctrl Pts',(-115.446738163493,100.524469125477,-67.2695400568307));
#13122=CARTESIAN_POINT('Ctrl Pts',(-114.405674258994,100.28486436115,-66.9123137382068));
#13123=CARTESIAN_POINT('Ctrl Pts',(-113.888815670701,100.22768844038,-66.6754382808512));
#13124=CARTESIAN_POINT('Ctrl Pts',(-113.435498258322,100.22768844038,-66.413715350786));
#13125=CARTESIAN_POINT('Ctrl Pts',(-113.045853744828,100.22768844038,-66.1887539860318));
#13126=CARTESIAN_POINT('Ctrl Pts',(-112.64222922698,100.270378061999,-65.9097091373666));
#13127=CARTESIAN_POINT('Ctrl Pts',(-111.934430306435,100.476843984392,-65.2895980494646));
#13128=CARTESIAN_POINT('Ctrl Pts',(-111.630654997402,100.641526829723,-64.9483785209879));
#13129=CARTESIAN_POINT('Ctrl Pts',(-111.2369795781,101.04252635731,-64.3493295404366));
#13130=CARTESIAN_POINT('Ctrl Pts',(-111.099937593526,101.284167988039,-64.0558123049316));
#13131=CARTESIAN_POINT('Ctrl Pts',(-110.986598478824,101.851747702853,-63.5337079966479));
#13132=CARTESIAN_POINT('Ctrl Pts',(-111.009713416376,102.178321465582,-63.3059402798856));
#13133=CARTESIAN_POINT('Ctrl Pts',(-111.191412176548,102.807744434161,-62.9912287955964));
#13134=CARTESIAN_POINT('Ctrl Pts',(-111.351088823113,103.136138059265,-62.8857591987216));
#13135=CARTESIAN_POINT('Ctrl Pts',(-111.565481622863,103.438089404292,-62.8444992851724));
#13136=CARTESIAN_POINT('Ctrl Pts',(-111.565481622863,103.438089404292,-62.8444992851724));
#13137=CARTESIAN_POINT('Ctrl Pts',(-111.575188933326,103.451761204159,-62.8426311124026));
#13138=CARTESIAN_POINT('Ctrl Pts',(-111.585003582125,103.465381199048,-62.8408869585381));
#13139=CARTESIAN_POINT('Ctrl Pts',(-111.823912628857,103.792091077249,-62.8018507603263));
#13140=CARTESIAN_POINT('Ctrl Pts',(-112.112006606371,104.073708899229,-62.8337382694769));
#13141=CARTESIAN_POINT('Ctrl Pts',(-112.759808395975,104.553028941455,-62.9926274651217));
#13142=CARTESIAN_POINT('Ctrl Pts',(-113.170797750173,104.759746443146,-63.1481468200871));
#13143=CARTESIAN_POINT('Ctrl Pts',(-114.013782161377,105.021576797287,-63.5341097697223));
#13144=CARTESIAN_POINT('Ctrl Pts',(-114.445853744829,105.077430701572,-63.7638828554352));
#13145=CARTESIAN_POINT('Ctrl Pts',(-115.288815670702,105.077430701572,-64.2505671502546));
#13146=CARTESIAN_POINT('Ctrl Pts',(-115.767594076423,105.002693000391,-64.5533994185862));
#13147=CARTESIAN_POINT('Ctrl Pts',(-116.652114853179,104.700016463066,-65.1817663880356));
#13148=CARTESIAN_POINT('Ctrl Pts',(-117.058123820432,104.473289105623,-65.5075087398144));
#13149=CARTESIAN_POINT('Ctrl Pts',(-117.59419825037,103.990784840806,-66.0388312545589));
#13150=CARTESIAN_POINT('Ctrl Pts',(-117.798111636135,103.73410733426,-66.281258295277));
#13151=CARTESIAN_POINT('Ctrl Pts',(-117.971447315925,103.296228661322,-66.6204521442011));
#13152=CARTESIAN_POINT('Ctrl Pts',(-118.007599536035,103.14149423203,-66.7297304001928));
#13153=CARTESIAN_POINT('Ctrl Pts',(-118.025761966741,102.824004944285,-66.9316462349407));
#13154=CARTESIAN_POINT('Ctrl Pts',(-118.007691799887,102.661241838733,-67.0242780679549));
#13155=CARTESIAN_POINT('Ctrl Pts',(-117.914598780889,102.338758161266,-67.1855199066884));
#13156=CARTESIAN_POINT('Ctrl Pts',(-117.839876304636,102.180078121956,-67.2536096461054));
#13157=CARTESIAN_POINT('Ctrl Pts',(-117.643713131067,101.879175318306,-67.3610917996573));
#13158=CARTESIAN_POINT('Ctrl Pts',(-117.522786130607,101.736775618063,-67.4007763629426));
#13159=CARTESIAN_POINT('Ctrl Pts',(-117.386134507204,101.60505912631,-67.4270749801282));
#13160=CARTESIAN_POINT('',(-106.165171981646,103.438089404295,-86.8623521842208));
#13161=CARTESIAN_POINT('',(-100.344519097302,101.605059126314,-82.2797764892636));
#13162=CARTESIAN_POINT('Ctrl Pts',(-106.165171981646,103.438089404295,-86.862352184219));
#13163=CARTESIAN_POINT('Ctrl Pts',(-106.14419730415,103.462308875692,-86.8634802540479));
#13164=CARTESIAN_POINT('Ctrl Pts',(-106.12282827633,103.486302635371,-86.8641514184887));
#13165=CARTESIAN_POINT('Ctrl Pts',(-105.818714172361,103.818683816975,-86.8673779259697));
#13166=CARTESIAN_POINT('Ctrl Pts',(-105.472391325601,104.085740432872,-86.7940722130298));
#13167=CARTESIAN_POINT('Ctrl Pts',(-104.731279077633,104.539153956812,-86.5696833263198));
#13168=CARTESIAN_POINT('Ctrl Pts',(-104.271314809741,104.741671619492,-86.3849512882693));
#13169=CARTESIAN_POINT('Ctrl Pts',(-103.33961664048,105.01118751589,-85.9511255373707));
#13170=CARTESIAN_POINT('Ctrl Pts',(-102.867626486497,105.077430701576,-85.7021134546504));
#13171=CARTESIAN_POINT('Ctrl Pts',(-102.441408937237,105.077430701576,-85.4560366378519));
#13172=CARTESIAN_POINT('Ctrl Pts',(-102.014157839508,105.077430701576,-85.2093631015665));
#13173=CARTESIAN_POINT('Ctrl Pts',(-101.56105927878,105.010210941309,-84.9242504184528));
#13174=CARTESIAN_POINT('Ctrl Pts',(-100.752419784988,104.696117862631,-84.3353138424256));
#13175=CARTESIAN_POINT('Ctrl Pts',(-100.397371710978,104.448780822016,-84.0310608152941));
#13176=CARTESIAN_POINT('Ctrl Pts',(-99.9882037851011,103.92339933994,-83.5499074785033));
#13177=CARTESIAN_POINT('Ctrl Pts',(-99.8584603905707,103.660815277971,-83.3448119619325));
#13178=CARTESIAN_POINT('Ctrl Pts',(-99.7452298798465,103.091082457567,-82.9637606339507));
#13179=CARTESIAN_POINT('Ctrl Pts',(-99.7621917782077,102.784236407494,-82.7872192164191));
#13180=CARTESIAN_POINT('Ctrl Pts',(-99.9262957445862,102.215763592511,-82.502982808928));
#13181=CARTESIAN_POINT('Ctrl Pts',(-100.082544658828,101.922589786887,-82.379514298611));
#13182=CARTESIAN_POINT('Ctrl Pts',(-100.312341841756,101.642706629092,-82.2911817419664));
#13183=CARTESIAN_POINT('Ctrl Pts',(-100.328291840436,101.623796748554,-82.2853723510623));
#13184=CARTESIAN_POINT('Ctrl Pts',(-100.344519097301,101.605059126315,-82.2797764892642));
#13185=CARTESIAN_POINT('Ctrl Pts',(-100.344519097301,101.605059126315,-82.2797764892642));
#13186=CARTESIAN_POINT('Ctrl Pts',(-100.550215520806,101.367541355351,-82.2088434432281));
#13187=CARTESIAN_POINT('Ctrl Pts',(-100.802602048525,101.15899254472,-82.1740857015096));
#13188=CARTESIAN_POINT('Ctrl Pts',(-101.47214666584,100.72565116497,-82.1694959867722));
#13189=CARTESIAN_POINT('Ctrl Pts',(-101.955786523501,100.527533200142,-82.2510215111824));
#13190=CARTESIAN_POINT('Ctrl Pts',(-102.926860882229,100.278935400847,-82.5586126482226));
#13191=CARTESIAN_POINT('Ctrl Pts',(-103.414157839508,100.227688440382,-82.784491970971));
#13192=CARTESIAN_POINT('Ctrl Pts',(-104.267626486497,100.227688440382,-83.2772423240549));
#13193=CARTESIAN_POINT('Ctrl Pts',(-104.705846427788,100.278428703028,-83.5847461309404));
#13194=CARTESIAN_POINT('Ctrl Pts',(-105.498304549662,100.491254479672,-84.2597427183605));
#13195=CARTESIAN_POINT('Ctrl Pts',(-105.853076223232,100.653134652889,-84.6266736743588));
#13196=CARTESIAN_POINT('Ctrl Pts',(-106.353797244182,101.032460766724,-85.2674323799564));
#13197=CARTESIAN_POINT('Ctrl Pts',(-106.557061980701,101.260971981571,-85.5885220082683));
#13198=CARTESIAN_POINT('Ctrl Pts',(-106.72625467127,101.679226130855,-86.024626674228));
#13199=CARTESIAN_POINT('Ctrl Pts',(-106.760576424903,101.831187432809,-86.1626137356242));
#13200=CARTESIAN_POINT('Ctrl Pts',(-106.774196861679,102.153837950614,-86.4089088160002));
#13201=CARTESIAN_POINT('Ctrl Pts',(-106.753460724005,102.324558208363,-86.5171780914983));
#13202=CARTESIAN_POINT('Ctrl Pts',(-106.652169358375,102.675441791642,-86.692619883138));
#13203=CARTESIAN_POINT('Ctrl Pts',(-106.572948453007,102.850982888141,-86.7574812847633));
#13204=CARTESIAN_POINT('Ctrl Pts',(-106.38376792248,103.164953280743,-86.8360360636708));
#13205=CARTESIAN_POINT('Ctrl Pts',(-106.28046465974,103.304960886828,-86.8561514599566));
#13206=CARTESIAN_POINT('Ctrl Pts',(-106.165171981646,103.438089404295,-86.862352184219));
#13207=CARTESIAN_POINT('',(-105.707515158216,101.445788778226,-60.813667453584));
#13208=CARTESIAN_POINT('',(-101.324821922316,103.6146594521,-56.8374045514775));
#13209=CARTESIAN_POINT('Ctrl Pts',(-105.707515158216,101.445788778225,-60.8136674535836));
#13210=CARTESIAN_POINT('Ctrl Pts',(-105.483577684551,101.227887906321,-60.8640309956986));
#13211=CARTESIAN_POINT('Ctrl Pts',(-105.222582053125,101.039304544329,-60.8807352012508));
#13212=CARTESIAN_POINT('Ctrl Pts',(-104.602960841079,100.67854055414,-60.8556299182567));
#13213=CARTESIAN_POINT('Ctrl Pts',(-104.1892589951,100.508020898325,-60.7865580098289));
#13214=CARTESIAN_POINT('Ctrl Pts',(-103.362197532696,100.282687776782,-60.5388045693685));
#13215=CARTESIAN_POINT('Ctrl Pts',(-102.949106981883,100.22768844038,-60.359394524506));
#13216=CARTESIAN_POINT('Ctrl Pts',(-102.587887471937,100.22768844038,-60.1508443432025));
#13217=CARTESIAN_POINT('Ctrl Pts',(-102.254878013721,100.22768844038,-59.9585812428588));
#13218=CARTESIAN_POINT('Ctrl Pts',(-101.918162195562,100.275039954704,-59.7132182406853));
#13219=CARTESIAN_POINT('Ctrl Pts',(-101.348088424631,100.488116881772,-59.166211609912));
#13220=CARTESIAN_POINT('Ctrl Pts',(-101.114826914581,100.65473625473,-58.8648160959221));
#13221=CARTESIAN_POINT('Ctrl Pts',(-100.809047976543,101.052694817512,-58.3193334032543));
#13222=CARTESIAN_POINT('Ctrl Pts',(-100.708587237918,101.302215526292,-58.04101395854));
#13223=CARTESIAN_POINT('Ctrl Pts',(-100.646124764096,101.871223563749,-57.5488477901271));
#13224=CARTESIAN_POINT('Ctrl Pts',(-100.683391349424,102.19108472861,-57.3355266127738));
#13225=CARTESIAN_POINT('Ctrl Pts',(-100.861743664517,102.808915271389,-57.0266113413844));
#13226=CARTESIAN_POINT('Ctrl Pts',(-101.013824739271,103.144973641637,-56.9119727511829));
#13227=CARTESIAN_POINT('Ctrl Pts',(-101.251985600091,103.511086021696,-56.8502538040771));
#13228=CARTESIAN_POINT('Ctrl Pts',(-101.287761408094,103.563290529642,-56.8430050519095));
#13229=CARTESIAN_POINT('Ctrl Pts',(-101.324821922315,103.614659452099,-56.8374045514776));
#13230=CARTESIAN_POINT('Ctrl Pts',(-101.324821922315,103.614659452099,-56.8374045514776));
#13231=CARTESIAN_POINT('Ctrl Pts',(-101.507571534895,103.867965453781,-56.8097878465912));
#13232=CARTESIAN_POINT('Ctrl Pts',(-101.722903603191,104.100150075329,-56.8237200261498));
#13233=CARTESIAN_POINT('Ctrl Pts',(-102.23560907329,104.537239540928,-56.9235644528227));
#13234=CARTESIAN_POINT('Ctrl Pts',(-102.577115242381,104.745590666186,-57.0374747177044));
#13235=CARTESIAN_POINT('Ctrl Pts',(-103.286625217418,105.015534918971,-57.3429707585513));
#13236=CARTESIAN_POINT('Ctrl Pts',(-103.654878013722,105.077430701572,-57.5337101122621));
#13237=CARTESIAN_POINT('Ctrl Pts',(-104.349106981883,105.077430701572,-57.9345233939092));
#13238=CARTESIAN_POINT('Ctrl Pts',(-104.725589216724,105.005615111484,-58.1773409020166));
#13239=CARTESIAN_POINT('Ctrl Pts',(-105.40533608587,104.720635512592,-58.6802507026948));
#13240=CARTESIAN_POINT('Ctrl Pts',(-105.708442531058,104.5080414619,-58.9408794643765));
#13241=CARTESIAN_POINT('Ctrl Pts',(-106.134628803274,104.039966782051,-59.3986735814598));
#13242=CARTESIAN_POINT('Ctrl Pts',(-106.301658407902,103.762601478164,-59.628755601445));
#13243=CARTESIAN_POINT('Ctrl Pts',(-106.466981515918,103.150363245665,-60.0574871392715));
#13244=CARTESIAN_POINT('Ctrl Pts',(-106.463597321879,102.815336528851,-60.256562220115));
#13245=CARTESIAN_POINT('Ctrl Pts',(-106.281537692062,102.184663471148,-60.5718987489666));
#13246=CARTESIAN_POINT('Ctrl Pts',(-106.096327018674,101.866378403104,-60.6994795605523));
#13247=CARTESIAN_POINT('Ctrl Pts',(-105.801011946827,101.53963142162,-60.790807331965));
#13248=CARTESIAN_POINT('Ctrl Pts',(-105.755075673419,101.492067221763,-60.8029710928037));
#13249=CARTESIAN_POINT('Ctrl Pts',(-105.707515158216,101.445788778225,-60.8136674535836));
#13250=CARTESIAN_POINT('',(-94.501534612098,103.614659452104,-80.2229951080884));
#13251=CARTESIAN_POINT('',(-90.1188413761952,101.445788778232,-76.2467322059816));
#13252=CARTESIAN_POINT('Ctrl Pts',(-94.5015346120983,103.614659452105,-80.222995108087));
#13253=CARTESIAN_POINT('Ctrl Pts',(-94.2999319259417,103.85835031517,-80.2346736634614));
#13254=CARTESIAN_POINT('Ctrl Pts',(-94.0660003649607,104.078184573876,-80.204501523942));
#13255=CARTESIAN_POINT('Ctrl Pts',(-93.506215357663,104.508041461903,-80.0757568941915));
#13256=CARTESIAN_POINT('Ctrl Pts',(-93.1289510064958,104.720635512595,-79.9435733934488));
#13257=CARTESIAN_POINT('Ctrl Pts',(-92.353544908723,105.005615111488,-79.6063502369639));
#13258=CARTESIAN_POINT('Ctrl Pts',(-91.9550176607982,105.077430701576,-79.4017158115723));
#13259=CARTESIAN_POINT('Ctrl Pts',(-91.5937981508529,105.077430701576,-79.1931656302689));
#13260=CARTESIAN_POINT('Ctrl Pts',(-91.2445310553966,105.077430701576,-78.9915161786881));
#13261=CARTESIAN_POINT('Ctrl Pts',(-90.8794457263923,105.009294935457,-78.75672916701));
#13262=CARTESIAN_POINT('Ctrl Pts',(-90.2394279750154,104.71379978534,-78.2726325195484));
#13263=CARTESIAN_POINT('Ctrl Pts',(-89.9651725619102,104.486205632632,-78.0225716794456));
#13264=CARTESIAN_POINT('Ctrl Pts',(-89.615152325688,103.992202355958,-77.5948073108704));
#13265=CARTESIAN_POINT('Ctrl Pts',(-89.4966157452444,103.711875068197,-77.3893068873646));
#13266=CARTESIAN_POINT('Ctrl Pts',(-89.4038756583846,103.11192693574,-77.0059525649689));
#13267=CARTESIAN_POINT('Ctrl Pts',(-89.4297352858526,102.792723417415,-76.8274306857825));
#13268=CARTESIAN_POINT('Ctrl Pts',(-89.5987392296941,102.207276582589,-76.5347072683697));
#13269=CARTESIAN_POINT('Ctrl Pts',(-89.7529823542094,101.902585866878,-76.4012820305381));
#13270=CARTESIAN_POINT('Ctrl Pts',(-90.0135013341837,101.566233275656,-76.2843454877329));
#13271=CARTESIAN_POINT('Ctrl Pts',(-90.0649390949408,101.505064596095,-76.2644831614807));
#13272=CARTESIAN_POINT('Ctrl Pts',(-90.1188413761922,101.445788778236,-76.2467322059833));
#13273=CARTESIAN_POINT('Ctrl Pts',(-90.1188413761922,101.445788778236,-76.2467322059833));
#13274=CARTESIAN_POINT('Ctrl Pts',(-90.3002565105157,101.246288307949,-76.1869890578052));
#13275=CARTESIAN_POINT('Ctrl Pts',(-90.5105127919593,101.068816696773,-76.1519939958911));
#13276=CARTESIAN_POINT('Ctrl Pts',(-91.0593017712658,100.696030871333,-76.1274842987972));
#13277=CARTESIAN_POINT('Ctrl Pts',(-91.4519661767371,100.513444242339,-76.1724547480489));
#13278=CARTESIAN_POINT('Ctrl Pts',(-92.2447448611874,100.279759997467,-76.3919616980159));
#13279=CARTESIAN_POINT('Ctrl Pts',(-92.6445310553966,100.227688440383,-76.5666450480926));
#13280=CARTESIAN_POINT('Ctrl Pts',(-93.3550176607982,100.227688440383,-76.9768446809768));
#13281=CARTESIAN_POINT('Ctrl Pts',(-93.7169365927499,100.282687776784,-77.2448865696132));
#13282=CARTESIAN_POINT('Ctrl Pts',(-94.3450280972656,100.508020898327,-77.8372660863158));
#13283=CARTESIAN_POINT('Ctrl Pts',(-94.6116970476415,100.678540554143,-78.1610064403122));
#13284=CARTESIAN_POINT('Ctrl Pts',(-94.9727271872904,101.071379412638,-78.7316542894256));
#13285=CARTESIAN_POINT('Ctrl Pts',(-95.1064606462321,101.310297639174,-79.0194069254365));
#13286=CARTESIAN_POINT('Ctrl Pts',(-95.2231499598568,101.866378403107,-79.5323746661135));
#13287=CARTESIAN_POINT('Ctrl Pts',(-95.2052670726821,102.184663471151,-79.7565622201121));
#13288=CARTESIAN_POINT('Ctrl Pts',(-95.0232074428643,102.815336528854,-80.0718987489636));
#13289=CARTESIAN_POINT('Ctrl Pts',(-94.8524954626127,103.150363245668,-80.174367087394));
#13290=CARTESIAN_POINT('Ctrl Pts',(-94.5857570770073,103.510107742139,-80.2161985863255));
#13291=CARTESIAN_POINT('Ctrl Pts',(-94.5443515978532,103.562903652559,-80.2205147813183));
#13292=CARTESIAN_POINT('Ctrl Pts',(-94.5015346120983,103.614659452105,-80.222995108087));
#13293=CARTESIAN_POINT('',(-94.2209929096256,101.354811290699,-54.2576156201439));
#13294=CARTESIAN_POINT('',(-90.5178421019398,103.716919354992,-50.5448617949466));
#13295=CARTESIAN_POINT('Ctrl Pts',(-94.2209929096261,101.354811290699,-54.2576156201434));
#13296=CARTESIAN_POINT('Ctrl Pts',(-94.0304505856294,101.165865871972,-54.3062458592498));
#13297=CARTESIAN_POINT('Ctrl Pts',(-93.8147279386984,100.999081132478,-54.3308652529223));
#13298=CARTESIAN_POINT('Ctrl Pts',(-93.2853347608051,100.664686636251,-54.335231850713));
#13299=CARTESIAN_POINT('Ctrl Pts',(-92.9240531847944,100.499668449628,-54.2909952556545));
#13300=CARTESIAN_POINT('Ctrl Pts',(-92.1976667058189,100.281331189612,-54.0944571890166));
#13301=CARTESIAN_POINT('Ctrl Pts',(-91.8328571384615,100.22768844038,-53.9414246850278));
#13302=CARTESIAN_POINT('Ctrl Pts',(-91.5141993333915,100.22768844038,-53.7574475154913));
#13303=CARTESIAN_POINT('Ctrl Pts',(-91.1998056536407,100.22768844038,-53.5759322398556));
#13304=CARTESIAN_POINT('Ctrl Pts',(-90.8886903708508,100.280334555034,-53.3396967948896));
#13305=CARTESIAN_POINT('Ctrl Pts',(-90.3733823362884,100.504055421459,-52.8139276391242));
#13306=CARTESIAN_POINT('Ctrl Pts',(-90.1688519647511,100.67573731595,-52.5249835715961));
#13307=CARTESIAN_POINT('Ctrl Pts',(-89.9037680431757,101.07557755986,-52.0026890248464));
#13308=CARTESIAN_POINT('Ctrl Pts',(-89.8203132445372,101.325643828305,-51.7350194741849));
#13309=CARTESIAN_POINT('Ctrl Pts',(-89.7787639540569,101.887795138889,-51.2622217134503));
#13310=CARTESIAN_POINT('Ctrl Pts',(-89.8201747804601,102.200227598979,-51.0575503555047));
#13311=CARTESIAN_POINT('Ctrl Pts',(-89.9932484568848,102.799772401019,-50.7577779544845));
#13312=CARTESIAN_POINT('Ctrl Pts',(-90.1366138563365,103.127423563352,-50.6424075012184));
#13313=CARTESIAN_POINT('Ctrl Pts',(-90.3868899039983,103.531966317969,-50.5657018885759));
#13314=CARTESIAN_POINT('Ctrl Pts',(-90.4505284239739,103.625948972014,-50.5527189917843));
#13315=CARTESIAN_POINT('Ctrl Pts',(-90.5178421019398,103.716919354992,-50.5448617949466));
#13316=CARTESIAN_POINT('Ctrl Pts',(-90.5178421019398,103.716919354992,-50.5448617949466));
#13317=CARTESIAN_POINT('Ctrl Pts',(-90.6677586076694,103.919522486378,-50.5273627734945));
#13318=CARTESIAN_POINT('Ctrl Pts',(-90.8363800498654,104.106877932436,-50.5357972502939));
#13319=CARTESIAN_POINT('Ctrl Pts',(-91.2761732604758,104.511610804944,-50.6070468270981));
#13320=CARTESIAN_POINT('Ctrl Pts',(-91.5920360022583,104.725595554037,-50.7031575728346));
#13321=CARTESIAN_POINT('Ctrl Pts',(-92.2536368706955,105.008647929721,-50.9755401075456));
#13322=CARTESIAN_POINT('Ctrl Pts',(-92.5998056536411,105.077430701572,-51.1510611092587));
#13323=CARTESIAN_POINT('Ctrl Pts',(-93.232857138462,105.077430701572,-51.5165535544309));
#13324=CARTESIAN_POINT('Ctrl Pts',(-93.5619700271323,105.00741652851,-51.7314145195672));
#13325=CARTESIAN_POINT('Ctrl Pts',(-94.1455671289826,104.731116876602,-52.1752710421669));
#13326=CARTESIAN_POINT('Ctrl Pts',(-94.3998110409153,104.525345718212,-52.4049023097321));
#13327=CARTESIAN_POINT('Ctrl Pts',(-94.768377540354,104.0613168212,-52.8259509372149));
#13328=CARTESIAN_POINT('Ctrl Pts',(-94.9105232806575,103.7725092302,-53.0468145506106));
#13329=CARTESIAN_POINT('Ctrl Pts',(-95.0354212815802,103.14720818058,-53.4590643079669));
#13330=CARTESIAN_POINT('Ctrl Pts',(-95.0172814114049,102.810893242388,-53.6509908389482));
#13331=CARTESIAN_POINT('Ctrl Pts',(-94.8377871142222,102.18910675761,-53.9618840813374));
#13332=CARTESIAN_POINT('Ctrl Pts',(-94.66647754768,101.869149596082,-54.0980936002161));
#13333=CARTESIAN_POINT('Ctrl Pts',(-94.365959399355,101.505588017214,-54.2160961273275));
#13334=CARTESIAN_POINT('Ctrl Pts',(-94.2953494579818,101.428544668509,-54.238638331267));
#13335=CARTESIAN_POINT('Ctrl Pts',(-94.2209929096261,101.354811290699,-54.2576156201434));
#13336=CARTESIAN_POINT('',(-83.0247832218288,103.716919354995,-73.6500196516034));
#13337=CARTESIAN_POINT('',(-79.3216324141422,101.354811290702,-69.9372658264059));
#13338=CARTESIAN_POINT('Ctrl Pts',(-83.0247832218292,103.716919354995,-73.6500196516021));
#13339=CARTESIAN_POINT('Ctrl Pts',(-82.8561874835582,103.929460895585,-73.6618384029087));
#13340=CARTESIAN_POINT('Ctrl Pts',(-82.6660644120803,104.123947093647,-73.6439402061671));
#13341=CARTESIAN_POINT('Ctrl Pts',(-82.1939330584629,104.523769595123,-73.5508930043753));
#13342=CARTESIAN_POINT('Ctrl Pts',(-81.8675496354975,104.73010984644,-73.445550762439));
#13343=CARTESIAN_POINT('Ctrl Pts',(-81.1904340361545,105.007198663853,-73.1618575252943));
#13344=CARTESIAN_POINT('Ctrl Pts',(-80.8392691645201,105.077430701576,-72.9840354250022));
#13345=CARTESIAN_POINT('Ctrl Pts',(-80.5201100123077,105.077430701576,-72.799768802558));
#13346=CARTESIAN_POINT('Ctrl Pts',(-80.2107074631239,105.077430701576,-72.6211351574988));
#13347=CARTESIAN_POINT('Ctrl Pts',(-79.8902928105569,105.010817414927,-72.4125520697033));
#13348=CARTESIAN_POINT('Ctrl Pts',(-79.3296459208272,104.735983399352,-71.9826313276384));
#13349=CARTESIAN_POINT('Ctrl Pts',(-79.0898300656876,104.528017888669,-71.760587957699));
#13350=CARTESIAN_POINT('Ctrl Pts',(-78.7510680657571,104.056494164301,-71.353383279585));
#13351=CARTESIAN_POINT('Ctrl Pts',(-78.6282785579301,103.763711210128,-71.1414137376349));
#13352=CARTESIAN_POINT('Ctrl Pts',(-78.5328756547392,103.137634877854,-70.745080894813));
#13353=CARTESIAN_POINT('Ctrl Pts',(-78.5604078289852,102.804749283705,-70.5600387968433));
#13354=CARTESIAN_POINT('Ctrl Pts',(-78.7363549099663,102.1952507163,-70.2552895131407));
#13355=CARTESIAN_POINT('Ctrl Pts',(-78.8964707374473,101.878104564589,-70.1153157381806));
#13356=CARTESIAN_POINT('Ctrl Pts',(-79.1804605765672,101.511189981574,-69.9855724361914));
#13357=CARTESIAN_POINT('Ctrl Pts',(-79.2490780626133,101.431324815456,-69.9596178450133));
#13358=CARTESIAN_POINT('Ctrl Pts',(-79.3216324141422,101.354811290702,-69.9372658264059));
#13359=CARTESIAN_POINT('Ctrl Pts',(-79.3216324141422,101.354811290702,-69.9372658264059));
#13360=CARTESIAN_POINT('Ctrl Pts',(-79.4994951487113,101.167242875335,-69.8824711646265));
#13361=CARTESIAN_POINT('Ctrl Pts',(-79.7016131069151,101.000214480644,-69.8498916678611));
#13362=CARTESIAN_POINT('Ctrl Pts',(-80.2057230797504,100.662451096332,-69.8278045615312));
#13363=CARTESIAN_POINT('Ctrl Pts',(-80.5536874604562,100.495779124926,-69.8625291904263));
#13364=CARTESIAN_POINT('Ctrl Pts',(-81.2563406796862,100.27868878512,-70.0464877548005));
#13365=CARTESIAN_POINT('Ctrl Pts',(-81.6107074631236,100.227688440383,-70.1962640269031));
#13366=CARTESIAN_POINT('Ctrl Pts',(-82.2392691645199,100.227688440383,-70.5591642944065));
#13367=CARTESIAN_POINT('Ctrl Pts',(-82.5546266768382,100.281496733901,-70.7990065603189));
#13368=CARTESIAN_POINT('Ctrl Pts',(-83.0885412363331,100.500470869914,-71.330731274177));
#13369=CARTESIAN_POINT('Ctrl Pts',(-83.3075860460983,100.665962481951,-71.6219894477902));
#13370=CARTESIAN_POINT('Ctrl Pts',(-83.6098374691532,101.054698410516,-72.1567503717173));
#13371=CARTESIAN_POINT('Ctrl Pts',(-83.7166215744316,101.303006298545,-72.4375565865388));
#13372=CARTESIAN_POINT('Ctrl Pts',(-83.7911705443989,101.870113330836,-72.9351916366745));
#13373=CARTESIAN_POINT('Ctrl Pts',(-83.7588055350932,102.189611224737,-73.1512430725076));
#13374=CARTESIAN_POINT('Ctrl Pts',(-83.5796024921405,102.810388775268,-73.4616318477727));
#13375=CARTESIAN_POINT('Ctrl Pts',(-83.4227987210069,103.14619075922,-73.5732303508662));
#13376=CARTESIAN_POINT('Ctrl Pts',(-83.1543827768569,103.546695163547,-73.6361875753525));
#13377=CARTESIAN_POINT('Ctrl Pts',(-83.0912106178557,103.633177136873,-73.6453630162586));
#13378=CARTESIAN_POINT('Ctrl Pts',(-83.0247832218292,103.716919354995,-73.6500196516021));
#13379=CARTESIAN_POINT('',(-79.2724338250639,100.514077983564,-46.3961169753473));
#13380=CARTESIAN_POINT('',(-82.9097405209592,104.714077983563,-45.6961169753459));
#13381=CARTESIAN_POINT('Ctrl Pts',(-79.2724338250643,100.514077983563,-46.3961169753468));
#13382=CARTESIAN_POINT('Ctrl Pts',(-79.1265511423845,100.610404906306,-46.2160498567682));
#13383=CARTESIAN_POINT('Ctrl Pts',(-79.0063377502804,100.729412390803,-46.0312428512855));
#13384=CARTESIAN_POINT('Ctrl Pts',(-78.7783882480642,101.056823805357,-45.5960981587349));
#13385=CARTESIAN_POINT('Ctrl Pts',(-78.6879980806413,101.308592332844,-45.3220312346838));
#13386=CARTESIAN_POINT('Ctrl Pts',(-78.637346637553,101.87720020589,-44.8375673373119));
#13387=CARTESIAN_POINT('Ctrl Pts',(-78.6768221832288,102.194506798829,-44.627746600585));
#13388=CARTESIAN_POINT('Ctrl Pts',(-78.8531987651598,102.805493201169,-44.3222533994151));
#13389=CARTESIAN_POINT('Ctrl Pts',(-79.001482969892,103.138605462875,-44.2068647088189));
#13390=CARTESIAN_POINT('Ctrl Pts',(-79.3969069246043,103.764324604201,-44.094165099005));
#13391=CARTESIAN_POINT('Ctrl Pts',(-79.6443545210792,104.056618970362,-44.0962005762319));
#13392=CARTESIAN_POINT('Ctrl Pts',(-80.1647562293486,104.52433820779,-44.1867417540882));
#13393=CARTESIAN_POINT('Ctrl Pts',(-80.4728761101798,104.731264722065,-44.2812762970742));
#13394=CARTESIAN_POINT('Ctrl Pts',(-81.1163900166925,105.008060588784,-44.5457120366282));
#13395=CARTESIAN_POINT('Ctrl Pts',(-81.4522447708355,105.077430701572,-44.7150138327633));
#13396=CARTESIAN_POINT('Ctrl Pts',(-82.0632775106341,105.077430701572,-45.0677937495697));
#13397=CARTESIAN_POINT('Ctrl Pts',(-82.3778245440648,105.008060588784,-45.2740016005717));
#13398=CARTESIAN_POINT('Ctrl Pts',(-82.7431217757092,104.824474558593,-45.5559387185791));
#13399=CARTESIAN_POINT('Ctrl Pts',(-82.8290587463787,104.772275635182,-45.6260680866036));
#13400=CARTESIAN_POINT('Ctrl Pts',(-82.9097405209591,104.714077983563,-45.6961169753458));
#13401=CARTESIAN_POINT('Ctrl Pts',(-82.9097405209591,104.714077983563,-45.6961169753458));
#13402=CARTESIAN_POINT('Ctrl Pts',(-83.0761634408585,104.594033237844,-45.8406073594606));
#13403=CARTESIAN_POINT('Ctrl Pts',(-83.2198007296756,104.447978167203,-45.9848429857255));
#13404=CARTESIAN_POINT('Ctrl Pts',(-83.5031306358671,104.056618970362,-46.3240660048471));
#13405=CARTESIAN_POINT('Ctrl Pts',(-83.6286172090919,103.764324604201,-46.5373441708864));
#13406=CARTESIAN_POINT('Ctrl Pts',(-83.7287284613526,103.138605462875,-46.936141165839));
#13407=CARTESIAN_POINT('Ctrl Pts',(-83.7029410263529,102.805493201169,-47.1222533994152));
#13408=CARTESIAN_POINT('Ctrl Pts',(-83.5265644444219,102.194506798829,-47.427746600585));
#13409=CARTESIAN_POINT('Ctrl Pts',(-83.3645921290135,101.87720020589,-47.5668437943321));
#13410=CARTESIAN_POINT('Ctrl Pts',(-82.9197083651289,101.308592332844,-47.7652103065652));
#13411=CARTESIAN_POINT('Ctrl Pts',(-82.6371643628521,101.056823805357,-47.8239635873502));
#13412=CARTESIAN_POINT('Ctrl Pts',(-82.0505767043741,100.665529520269,-47.8480598380025));
#13413=CARTESIAN_POINT('Ctrl Pts',(-81.7069979829943,100.499547348265,-47.8149418084238));
#13414=CARTESIAN_POINT('Ctrl Pts',(-81.0131896142114,100.280826524207,-47.637618632861));
#13415=CARTESIAN_POINT('Ctrl Pts',(-80.6632775106336,100.227688440379,-47.4926648801669));
#13416=CARTESIAN_POINT('Ctrl Pts',(-80.3577611407344,100.227688440379,-47.3162749217637));
#13417=CARTESIAN_POINT('Ctrl Pts',(-80.0522447708351,100.227688440379,-47.1398849633606));
#13418=CARTESIAN_POINT('Ctrl Pts',(-79.7517550868392,100.280826524207,-46.9093290689175));
#13419=CARTESIAN_POINT('Ctrl Pts',(-79.4198158701761,100.42589403654,-46.5696141741228));
#13420=CARTESIAN_POINT('Ctrl Pts',(-79.3431576996741,100.467378724402,-46.4834134527748));
#13421=CARTESIAN_POINT('Ctrl Pts',(-79.2724338250643,100.514077983563,-46.3961169753468));
#13422=CARTESIAN_POINT('',(-68.2116924394259,104.714077983566,-65.5538830246524));
#13423=CARTESIAN_POINT('',(-71.8489991353209,100.514077983566,-64.8538830246516));
#13424=CARTESIAN_POINT('Ctrl Pts',(-68.2116924394265,104.714077983567,-65.5538830246511));
#13425=CARTESIAN_POINT('Ctrl Pts',(-68.0452695195272,104.594033237848,-65.4093926405365));
#13426=CARTESIAN_POINT('Ctrl Pts',(-67.9016322307103,104.447978167207,-65.2651570142717));
#13427=CARTESIAN_POINT('Ctrl Pts',(-67.6183023245187,104.056618970366,-64.9259339951503));
#13428=CARTESIAN_POINT('Ctrl Pts',(-67.4928157512939,103.764324604205,-64.7126558291111));
#13429=CARTESIAN_POINT('Ctrl Pts',(-67.3927044990331,103.138605462879,-64.3138588341587));
#13430=CARTESIAN_POINT('Ctrl Pts',(-67.4184919340327,102.805493201172,-64.1277466005826));
#13431=CARTESIAN_POINT('Ctrl Pts',(-67.5948685159636,102.194506798833,-63.8222533994129));
#13432=CARTESIAN_POINT('Ctrl Pts',(-67.7568408313719,101.877200205893,-63.683156205666));
#13433=CARTESIAN_POINT('Ctrl Pts',(-68.2017245952565,101.308592332847,-63.484789693433));
#13434=CARTESIAN_POINT('Ctrl Pts',(-68.4842685975332,101.056823805361,-63.4260364126481));
#13435=CARTESIAN_POINT('Ctrl Pts',(-69.0708562560112,100.665529520272,-63.4019401619959));
#13436=CARTESIAN_POINT('Ctrl Pts',(-69.4144349773908,100.499547348269,-63.4350581915746));
#13437=CARTESIAN_POINT('Ctrl Pts',(-70.1082433461736,100.28082652421,-63.6123813671375));
#13438=CARTESIAN_POINT('Ctrl Pts',(-70.4581554497515,100.227688440383,-63.7573351198316));
#13439=CARTESIAN_POINT('Ctrl Pts',(-71.0691881895501,100.227688440383,-64.110115036638));
#13440=CARTESIAN_POINT('Ctrl Pts',(-71.369677873546,100.28082652421,-64.340670931081));
#13441=CARTESIAN_POINT('Ctrl Pts',(-71.701617090209,100.425894036543,-64.6803858258755));
#13442=CARTESIAN_POINT('Ctrl Pts',(-71.7782752607111,100.467378724405,-64.7665865472236));
#13443=CARTESIAN_POINT('Ctrl Pts',(-71.8489991353208,100.514077983566,-64.8538830246515));
#13444=CARTESIAN_POINT('Ctrl Pts',(-71.8489991353208,100.514077983566,-64.8538830246515));
#13445=CARTESIAN_POINT('Ctrl Pts',(-71.9948818180007,100.61040490631,-65.0339501432301));
#13446=CARTESIAN_POINT('Ctrl Pts',(-72.1150952101049,100.729412390806,-65.2187571487129));
#13447=CARTESIAN_POINT('Ctrl Pts',(-72.3430447123212,101.056823805361,-65.6539018412633));
#13448=CARTESIAN_POINT('Ctrl Pts',(-72.4334348797441,101.308592332847,-65.9279687653144));
#13449=CARTESIAN_POINT('Ctrl Pts',(-72.4840863228325,101.877200205893,-66.4124326626861));
#13450=CARTESIAN_POINT('Ctrl Pts',(-72.4446107771567,102.194506798833,-66.622253399413));
#13451=CARTESIAN_POINT('Ctrl Pts',(-72.2682341952258,102.805493201172,-66.9277466005826));
#13452=CARTESIAN_POINT('Ctrl Pts',(-72.1199499904937,103.138605462879,-67.0431352911788));
#13453=CARTESIAN_POINT('Ctrl Pts',(-71.7245260357815,103.764324604205,-67.1558349009925));
#13454=CARTESIAN_POINT('Ctrl Pts',(-71.4770784393067,104.056618970366,-67.1537994237656));
#13455=CARTESIAN_POINT('Ctrl Pts',(-70.9566767310373,104.524338207794,-67.0632582459091));
#13456=CARTESIAN_POINT('Ctrl Pts',(-70.6485568502061,104.731264722069,-66.968723702923));
#13457=CARTESIAN_POINT('Ctrl Pts',(-70.0050429436934,105.008060588788,-66.7042879633689));
#13458=CARTESIAN_POINT('Ctrl Pts',(-69.6691881895505,105.077430701576,-66.5349861672338));
#13459=CARTESIAN_POINT('Ctrl Pts',(-69.3636718196512,105.077430701576,-66.3585962088306));
#13460=CARTESIAN_POINT('Ctrl Pts',(-69.0581554497519,105.077430701576,-66.1822062504275));
#13461=CARTESIAN_POINT('Ctrl Pts',(-68.7436084163211,105.008060588788,-65.9759983994254));
#13462=CARTESIAN_POINT('Ctrl Pts',(-68.3783111846766,104.824474558597,-65.694061281418));
#13463=CARTESIAN_POINT('Ctrl Pts',(-68.292374214007,104.772275635186,-65.6239319133934));
#13464=CARTESIAN_POINT('Ctrl Pts',(-68.2116924394265,104.714077983567,-65.5538830246511));
#13465=CARTESIAN_POINT('',(-112.569378637745,121.956851469395,-75.7699408736866));
#13466=CARTESIAN_POINT('',(-105.161274966764,121.956851469395,-73.9369105957041));
#13467=CARTESIAN_POINT('Ctrl Pts',(-112.569378637745,121.956851469395,-75.7699408736867));
#13468=CARTESIAN_POINT('Ctrl Pts',(-112.569272008943,121.95672834506,-75.7681386924676));
#13469=CARTESIAN_POINT('Ctrl Pts',(-112.569163342679,121.956605035935,-75.7663364623398));
#13470=CARTESIAN_POINT('Ctrl Pts',(-112.545386428826,121.930081208774,-75.3792452325324));
#13471=CARTESIAN_POINT('Ctrl Pts',(-112.425619842949,121.895265649918,-74.9910716591131));
#13472=CARTESIAN_POINT('Ctrl Pts',(-112.050450493293,121.820378366244,-74.1810533701236));
#13473=CARTESIAN_POINT('Ctrl Pts',(-111.722843184654,121.775514411454,-73.719515362228));
#13474=CARTESIAN_POINT('Ctrl Pts',(-110.943904850608,121.712442638456,-72.9082742376171));
#13475=CARTESIAN_POINT('Ctrl Pts',(-110.491771010159,121.694880858045,-72.5592922284894));
#13476=CARTESIAN_POINT('Ctrl Pts',(-110.03845359778,121.694880858045,-72.2975692984242));
#13477=CARTESIAN_POINT('Ctrl Pts',(-109.648809084286,121.694880858045,-72.07260793367));
#13478=CARTESIAN_POINT('Ctrl Pts',(-109.196813666427,121.708045140711,-71.8773439414328));
#13479=CARTESIAN_POINT('Ctrl Pts',(-108.262263007713,121.76340957246,-71.6499783847423));
#13480=CARTESIAN_POINT('Ctrl Pts',(-107.779465090809,121.805444228819,-71.6188351088017));
#13481=CARTESIAN_POINT('Ctrl Pts',(-106.970686338396,121.883764743458,-71.7387661915901));
#13482=CARTESIAN_POINT('Ctrl Pts',(-106.589756165829,121.923740934709,-71.8676756890549));
#13483=CARTESIAN_POINT('Ctrl Pts',(-105.93403329749,121.982452032228,-72.2850075992705));
#13484=CARTESIAN_POINT('Ctrl Pts',(-105.659130074434,121.999999999998,-72.5734224782579));
#13485=CARTESIAN_POINT('Ctrl Pts',(-105.295732554092,121.999999999998,-73.2028454468363));
#13486=CARTESIAN_POINT('Ctrl Pts',(-105.184827334639,121.984047401261,-73.5660373895111));
#13487=CARTESIAN_POINT('Ctrl Pts',(-105.161274966764,121.956851469395,-73.936910595704));
#13488=CARTESIAN_POINT('Ctrl Pts',(-105.161274966764,121.956851469395,-73.936910595704));
#13489=CARTESIAN_POINT('Ctrl Pts',(-105.160208558995,121.955620087771,-73.9537030502982));
#13490=CARTESIAN_POINT('Ctrl Pts',(-105.159312222542,121.954368073319,-73.9705108670905));
#13491=CARTESIAN_POINT('Ctrl Pts',(-105.141806095166,121.923740934709,-74.3755987782653));
#13492=CARTESIAN_POINT('Ctrl Pts',(-105.220632281856,121.883764743458,-74.7699487335092));
#13493=CARTESIAN_POINT('Ctrl Pts',(-105.521158293664,121.805444228818,-75.5303372205339));
#13494=CARTESIAN_POINT('Ctrl Pts',(-105.789528120238,121.763409572459,-75.9328808434969));
#13495=CARTESIAN_POINT('Ctrl Pts',(-106.453707797634,121.708045140711,-76.628542676721));
#13496=CARTESIAN_POINT('Ctrl Pts',(-106.848809084286,121.694880858045,-76.9223501948628));
#13497=CARTESIAN_POINT('Ctrl Pts',(-107.691771010159,121.694880858045,-77.4090344896822));
#13498=CARTESIAN_POINT('Ctrl Pts',(-108.220065215752,121.712442638456,-77.6261028768581));
#13499=CARTESIAN_POINT('Ctrl Pts',(-109.312089805283,121.775514411454,-77.895062699818));
#13500=CARTESIAN_POINT('Ctrl Pts',(-109.875597099252,121.820378366244,-77.948009947617));
#13501=CARTESIAN_POINT('Ctrl Pts',(-110.764678189875,121.895265649918,-77.8679069906454));
#13502=CARTESIAN_POINT('Ctrl Pts',(-111.160729658472,121.930081208774,-77.7775411098295));
#13503=CARTESIAN_POINT('Ctrl Pts',(-111.678984353092,121.96968170959,-77.5193177005707));
#13504=CARTESIAN_POINT('Ctrl Pts',(-111.839559773292,121.980744602752,-77.4130886523666));
#13505=CARTESIAN_POINT('Ctrl Pts',(-112.11953636853,121.995916933756,-77.161529052004));
#13506=CARTESIAN_POINT('Ctrl Pts',(-112.238887146792,121.999999999998,-77.016140826053));
#13507=CARTESIAN_POINT('Ctrl Pts',(-112.425073184787,121.999999999998,-76.693657148586));
#13508=CARTESIAN_POINT('Ctrl Pts',(-112.491307692741,121.995916933756,-76.5176022296746));
#13509=CARTESIAN_POINT('Ctrl Pts',(-112.568812151847,121.980815574618,-76.1510781390455));
#13510=CARTESIAN_POINT('Ctrl Pts',(-112.580669535468,121.969889075075,-75.9607734026514));
#13511=CARTESIAN_POINT('Ctrl Pts',(-112.569378637745,121.956851469395,-75.7699408736867));
#13512=CARTESIAN_POINT('',(-101.043673435707,121.93955176967,-68.8916782754278));
#13513=CARTESIAN_POINT('',(-94.7826830987082,121.939551769669,-68.1687213841338));
#13514=CARTESIAN_POINT('Ctrl Pts',(-101.043673435707,121.93955176967,-68.8916782754277));
#13515=CARTESIAN_POINT('Ctrl Pts',(-101.030778440127,121.913761778509,-68.5765055229452));
#13516=CARTESIAN_POINT('Ctrl Pts',(-100.960164861362,121.882510881795,-68.2634583404383));
#13517=CARTESIAN_POINT('Ctrl Pts',(-100.712810634339,121.813417983957,-67.5935677254039));
#13518=CARTESIAN_POINT('Ctrl Pts',(-100.483220636953,121.771343589081,-67.2056047409378));
#13519=CARTESIAN_POINT('Ctrl Pts',(-99.9029587467504,121.711697111731,-66.5303819021385));
#13520=CARTESIAN_POINT('Ctrl Pts',(-99.5520623213409,121.694880858045,-66.2432484721442));
#13521=CARTESIAN_POINT('Ctrl Pts',(-99.1908428113955,121.694880858045,-66.0346982908408));
#13522=CARTESIAN_POINT('Ctrl Pts',(-98.8578333531796,121.694880858045,-65.8424351904971));
#13523=CARTESIAN_POINT('Ctrl Pts',(-98.4675142149001,121.709425126322,-65.6899158622252));
#13524=CARTESIAN_POINT('Ctrl Pts',(-97.6636618634519,121.766292452039,-65.5478256106297));
#13525=CARTESIAN_POINT('Ctrl Pts',(-97.2499629860219,121.808024204338,-65.5589567845263));
#13526=CARTESIAN_POINT('Ctrl Pts',(-96.532228635356,121.885750778307,-65.7270017969835));
#13527=CARTESIAN_POINT('Ctrl Pts',(-96.1806212553106,121.926229231586,-65.8836810953591));
#13528=CARTESIAN_POINT('Ctrl Pts',(-95.5755231979279,121.983802794611,-66.3313873276683));
#13529=CARTESIAN_POINT('Ctrl Pts',(-95.3217546974658,121.999999999998,-66.6221537056877));
#13530=CARTESIAN_POINT('Ctrl Pts',(-94.9650500672789,121.999999999998,-67.2399842484664));
#13531=CARTESIAN_POINT('Ctrl Pts',(-94.8401232475787,121.983802794611,-67.6051374055565));
#13532=CARTESIAN_POINT('Ctrl Pts',(-94.7903548426391,121.950162492739,-68.0421265757317));
#13533=CARTESIAN_POINT('Ctrl Pts',(-94.7854013049624,121.944988182178,-68.1054231196404));
#13534=CARTESIAN_POINT('Ctrl Pts',(-94.7826830987084,121.93955176967,-68.168721384132));
#13535=CARTESIAN_POINT('Ctrl Pts',(-94.7826830987083,121.93955176967,-68.168721384132));
#13536=CARTESIAN_POINT('Ctrl Pts',(-94.7692793143766,121.912744201006,-68.4808523287743));
#13537=CARTESIAN_POINT('Ctrl Pts',(-94.8123721828179,121.87944427626,-68.7931115535356));
#13538=CARTESIAN_POINT('Ctrl Pts',(-95.0083986686057,121.808024204338,-69.4414600707244));
#13539=CARTESIAN_POINT('Ctrl Pts',(-95.2056082279524,121.766292452039,-69.8052993950442));
#13540=CARTESIAN_POINT('Ctrl Pts',(-95.7305881711883,121.709425126322,-70.4304108264924));
#13541=CARTESIAN_POINT('Ctrl Pts',(-96.0578333531797,121.694880858045,-70.6921774516898));
#13542=CARTESIAN_POINT('Ctrl Pts',(-96.7520623213409,121.694880858045,-71.0929907333369));
#13543=CARTESIAN_POINT('Ctrl Pts',(-97.1761753786965,121.711697111731,-71.2533092368416));
#13544=CARTESIAN_POINT('Ctrl Pts',(-98.0510664554135,121.771343589081,-71.4182193552053));
#13545=CARTESIAN_POINT('Ctrl Pts',(-98.5018472543822,121.813417983957,-71.4230686331636));
#13546=CARTESIAN_POINT('Ctrl Pts',(-99.2682419576485,121.888653805311,-71.2916044625037));
#13547=CARTESIAN_POINT('Ctrl Pts',(-99.6421808158843,121.927100882661,-71.163309142685));
#13548=CARTESIAN_POINT('Ctrl Pts',(-100.289083992022,121.983258351228,-70.7579195346131));
#13549=CARTESIAN_POINT('Ctrl Pts',(-100.561342752554,121.999999999998,-70.4795670133904));
#13550=CARTESIAN_POINT('Ctrl Pts',(-100.92546201219,121.999999999998,-69.8488939556873));
#13551=CARTESIAN_POINT('Ctrl Pts',(-101.03039298651,121.983258351228,-69.4739346920516));
#13552=CARTESIAN_POINT('Ctrl Pts',(-101.046625787479,121.950260836241,-69.0256457187578));
#13553=CARTESIAN_POINT('Ctrl Pts',(-101.046412113711,121.945029125677,-68.9586156139657));
#13554=CARTESIAN_POINT('Ctrl Pts',(-101.043673435707,121.93955176967,-68.8916782754277));
#13555=CARTESIAN_POINT('',(-89.6457108608091,121.928269354306,-62.1822365876521));
#13556=CARTESIAN_POINT('',(-83.8969144629603,121.928269354306,-62.0126448588956));
#13557=CARTESIAN_POINT('Ctrl Pts',(-89.6457108608091,121.928269354306,-62.1822365876521));
#13558=CARTESIAN_POINT('Ctrl Pts',(-89.640048215299,121.903866743648,-61.9118469440624));
#13559=CARTESIAN_POINT('Ctrl Pts',(-89.5938110699338,121.875525701933,-61.6447310127997));
#13560=CARTESIAN_POINT('Ctrl Pts',(-89.4114212651875,121.810267922929,-61.0498367272997));
#13561=CARTESIAN_POINT('Ctrl Pts',(-89.2283577823594,121.76941928365,-60.6962570673076));
#13562=CARTESIAN_POINT('Ctrl Pts',(-88.7408793475757,121.711304602249,-60.0841026261431));
#13563=CARTESIAN_POINT('Ctrl Pts',(-88.4363138250625,121.694880858045,-59.8255680855737));
#13564=CARTESIAN_POINT('Ctrl Pts',(-88.11715467285,121.694880858045,-59.6413014631295));
#13565=CARTESIAN_POINT('Ctrl Pts',(-87.8077521236662,121.694880858045,-59.4626678180703));
#13566=CARTESIAN_POINT('Ctrl Pts',(-87.4431698769551,121.710493799957,-59.3305852473804));
#13567=CARTESIAN_POINT('Ctrl Pts',(-86.6945172380366,121.768237475725,-59.2263000150256));
#13568=CARTESIAN_POINT('Ctrl Pts',(-86.3103592215609,121.809531015002,-59.2542646021946));
#13569=CARTESIAN_POINT('Ctrl Pts',(-85.6299700128694,121.886577617489,-59.4387756069027));
#13570=CARTESIAN_POINT('Ctrl Pts',(-85.2887695763051,121.927161354661,-59.6051048904537));
#13571=CARTESIAN_POINT('Ctrl Pts',(-84.7006180249038,121.984260557561,-60.0622377416933));
#13572=CARTESIAN_POINT('Ctrl Pts',(-84.4534935750556,121.999999999998,-60.35291487129));
#13573=CARTESIAN_POINT('Ctrl Pts',(-84.1015994130934,121.999999999998,-60.9624134386954));
#13574=CARTESIAN_POINT('Ctrl Pts',(-83.9734278594876,121.98426055756,-61.3217680549585));
#13575=CARTESIAN_POINT('Ctrl Pts',(-83.9077720873625,121.947439165029,-61.7976287162892));
#13576=CARTESIAN_POINT('Ctrl Pts',(-83.8992173832946,121.938193561674,-61.9053402793198));
#13577=CARTESIAN_POINT('Ctrl Pts',(-83.8969144629603,121.928269354306,-62.0126448588956));
#13578=CARTESIAN_POINT('Ctrl Pts',(-83.8969144629603,121.928269354306,-62.0126448588956));
#13579=CARTESIAN_POINT('Ctrl Pts',(-83.8912689889189,121.903940742393,-62.2756957380355));
#13580=CARTESIAN_POINT('Ctrl Pts',(-83.9241062924374,121.875500673982,-62.5363189359234));
#13581=CARTESIAN_POINT('Ctrl Pts',(-84.0785731934348,121.809531015002,-63.1198313945313));
#13582=CARTESIAN_POINT('Ctrl Pts',(-84.246434158778,121.768237475725,-63.4665042894511));
#13583=CARTESIAN_POINT('Ctrl Pts',(-84.7110741386961,121.710493799957,-64.0627138771875));
#13584=CARTESIAN_POINT('Ctrl Pts',(-85.0077521236662,121.694880858045,-64.3124100792631));
#13585=CARTESIAN_POINT('Ctrl Pts',(-85.6363138250625,121.694880858045,-64.6753103467665));
#13586=CARTESIAN_POINT('Ctrl Pts',(-86.012494066208,121.711304602249,-64.8098045560952));
#13587=CARTESIAN_POINT('Ctrl Pts',(-86.7863745806878,121.76941928365,-64.9258960438327));
#13588=CARTESIAN_POINT('Ctrl Pts',(-87.1841152899164,121.810267922929,-64.907643840471));
#13589=CARTESIAN_POINT('Ctrl Pts',(-87.8886874328802,121.886091946244,-64.7455648365782));
#13590=CARTESIAN_POINT('Ctrl Pts',(-88.245336954858,121.9263037894,-64.5935914546221));
#13591=CARTESIAN_POINT('Ctrl Pts',(-88.8607180558249,121.983695909948,-64.1544777755007));
#13592=CARTESIAN_POINT('Ctrl Pts',(-89.1191660952628,121.999999999998,-63.866826235406));
#13593=CARTESIAN_POINT('Ctrl Pts',(-89.4775721811683,121.999999999998,-63.2460486848757));
#13594=CARTESIAN_POINT('Ctrl Pts',(-89.5974617026091,121.983695909948,-62.8784003471169));
#13595=CARTESIAN_POINT('Ctrl Pts',(-89.6440171485706,121.946889139357,-62.3958111209995));
#13596=CARTESIAN_POINT('Ctrl Pts',(-89.6479419658163,121.937884080627,-62.2887711900116));
#13597=CARTESIAN_POINT('Ctrl Pts',(-89.6457108608091,121.928269354306,-62.1822365876521));
#13598=CARTESIAN_POINT('',(-75.5607164801933,121.77184403287,-52.8249999999979));
#13599=CARTESIAN_POINT('',(-75.5607164801932,121.77184403287,-58.4249999999981));
#13600=CARTESIAN_POINT('Ctrl Pts',(-75.5607164801933,121.77184403287,-52.8249999999979));
#13601=CARTESIAN_POINT('Ctrl Pts',(-75.31087199813,121.795561855846,-52.8249999999979));
#13602=CARTESIAN_POINT('Ctrl Pts',(-75.0641712044988,121.822609441991,-52.8592756004775));
#13603=CARTESIAN_POINT('Ctrl Pts',(-74.4972946958141,121.886557224277,-53.0111697031877));
#13604=CARTESIAN_POINT('Ctrl Pts',(-74.1537701819123,121.927083062952,-53.1755443283788));
#13605=CARTESIAN_POINT('Ctrl Pts',(-73.561230066802,121.984194331231,-53.6296591429951));
#13606=CARTESIAN_POINT('Ctrl Pts',(-73.3122219315277,121.999999999998,-53.9195067988283));
#13607=CARTESIAN_POINT('Ctrl Pts',(-72.9594687676658,121.999999999998,-54.5304932011677));
#13608=CARTESIAN_POINT('Ctrl Pts',(-72.8329574021241,121.984194331231,-54.8910643999808));
#13609=CARTESIAN_POINT('Ctrl Pts',(-72.7359524939867,121.927083062952,-55.6312765997358));
#13610=CARTESIAN_POINT('Ctrl Pts',(-72.7653621497846,121.886557224277,-56.010964868193));
#13611=CARTESIAN_POINT('Ctrl Pts',(-72.9468930668116,121.810132271938,-56.6884474736823));
#13612=CARTESIAN_POINT('Ctrl Pts',(-73.1112681701126,121.769187929666,-57.0319552746733));
#13613=CARTESIAN_POINT('Ctrl Pts',(-73.5653642866542,121.711112887006,-57.6244722503148));
#13614=CARTESIAN_POINT('Ctrl Pts',(-73.855200110294,121.694880858045,-57.8734811721914));
#13615=CARTESIAN_POINT('Ctrl Pts',(-74.4662328500925,121.694880858045,-58.2262610889977));
#13616=CARTESIAN_POINT('Ctrl Pts',(-74.8267988140265,121.711112887006,-58.3527618142583));
#13617=CARTESIAN_POINT('Ctrl Pts',(-75.3177281966151,121.749631404864,-58.4170976637661));
#13618=CARTESIAN_POINT('Ctrl Pts',(-75.4395919608409,121.760345640413,-58.4249999999981));
#13619=CARTESIAN_POINT('Ctrl Pts',(-75.560716480193,121.77184403287,-58.4249999999981));
#13620=CARTESIAN_POINT('Ctrl Pts',(-75.560716480193,121.77184403287,-58.4249999999981));
#13621=CARTESIAN_POINT('Ctrl Pts',(-75.8105609622564,121.795561855846,-58.4249999999981));
#13622=CARTESIAN_POINT('Ctrl Pts',(-76.0572617558877,121.822609441991,-58.3907243995186));
#13623=CARTESIAN_POINT('Ctrl Pts',(-76.6241382645725,121.886557224277,-58.2388302968083));
#13624=CARTESIAN_POINT('Ctrl Pts',(-76.9676627784743,121.927083062952,-58.0744556716172));
#13625=CARTESIAN_POINT('Ctrl Pts',(-77.5602028935846,121.984194331231,-57.620340857001));
#13626=CARTESIAN_POINT('Ctrl Pts',(-77.8092110288589,121.999999999998,-57.3304932011678));
#13627=CARTESIAN_POINT('Ctrl Pts',(-78.1619641927208,121.999999999998,-56.7195067988283));
#13628=CARTESIAN_POINT('Ctrl Pts',(-78.2884755582626,121.984194331231,-56.3589356000152));
#13629=CARTESIAN_POINT('Ctrl Pts',(-78.3854804663999,121.927083062952,-55.6187234002602));
#13630=CARTESIAN_POINT('Ctrl Pts',(-78.356070810602,121.886557224277,-55.239035131803));
#13631=CARTESIAN_POINT('Ctrl Pts',(-78.174539893575,121.810132271938,-54.5615525263137));
#13632=CARTESIAN_POINT('Ctrl Pts',(-78.010164790274,121.769187929666,-54.2180447253227));
#13633=CARTESIAN_POINT('Ctrl Pts',(-77.5560686737324,121.711112887006,-53.6255277496812));
#13634=CARTESIAN_POINT('Ctrl Pts',(-77.2662328500926,121.694880858045,-53.3765188278046));
#13635=CARTESIAN_POINT('Ctrl Pts',(-76.9607164801934,121.694880858045,-53.2001288694015));
#13636=CARTESIAN_POINT('Ctrl Pts',(-76.6552001102941,121.694880858045,-53.0237389109983));
#13637=CARTESIAN_POINT('Ctrl Pts',(-76.2946341463601,121.711112887006,-52.8972381857377));
#13638=CARTESIAN_POINT('Ctrl Pts',(-75.8037047637714,121.749631404864,-52.8329023362299));
#13639=CARTESIAN_POINT('Ctrl Pts',(-75.6818409995455,121.760345640413,-52.8249999999979));
#13640=CARTESIAN_POINT('Ctrl Pts',(-75.5607164801933,121.77184403287,-52.8249999999979));
#13641=CARTESIAN_POINT('Origin',(-115.614391405224,109.,-78.7499999999976));
#13642=CARTESIAN_POINT('Origin',(-111.692877174869,125.221825406948,-76.4859127034721));
#13643=CARTESIAN_POINT('',(-109.047125863805,127.513113254426,-76.4859127034721));
#13644=CARTESIAN_POINT('Origin',(-111.692877174869,125.221825406948,-76.4859127034721));
#13645=CARTESIAN_POINT('',(-109.576276126018,127.054855684931,-76.4859127034722));
#13646=CARTESIAN_POINT('Origin',(-111.692877174869,125.221825406948,-76.4859127034722));
#13647=CARTESIAN_POINT('Origin',(-111.692877174869,125.221825406948,-76.4859127034721));
#13648=CARTESIAN_POINT('',(-109.047125863805,127.513113254426,-76.4859127034721));
#13649=CARTESIAN_POINT('Origin',(-75.5607164801933,112.,-55.624999999998));
#13650=CARTESIAN_POINT('',(-75.5607164801933,112.,-58.4249999999981));
#13651=CARTESIAN_POINT('Origin',(-84.3932587967998,111.68028146752,-60.7244706841197));
#13652=CARTESIAN_POINT('',(-81.6657313432502,112.313206415782,-60.7244706841197));
#13653=CARTESIAN_POINT('Origin',(-93.3501356426365,112.813466520527,-65.8957259421618));
#13654=CARTESIAN_POINT('',(-90.8457395078369,114.065664587927,-65.8957259421618));
#13655=CARTESIAN_POINT('Origin',(-103.119663075128,115.322330470337,-71.5361652351663));
#13656=CARTESIAN_POINT('',(-101.003062026277,117.155360748319,-71.5361652351663));
#13657=CARTESIAN_POINT('Origin',(-84.2209705180366,98.999999999999,-40.6249999999996));
#13658=CARTESIAN_POINT('',(-86.8190467293899,101.999999999999,-40.1249999999996));
#13659=CARTESIAN_POINT('Origin',(-84.2209705180366,98.999999999999,-40.6249999999996));
#13660=CARTESIAN_POINT('',(-86.4942872029708,101.624999999999,-40.1874999999995));
#13661=CARTESIAN_POINT('Origin',(-84.2209705180366,98.999999999999,-40.6249999999996));
#13662=CARTESIAN_POINT('Origin',(-26.1968246264604,166.000512499998,-141.125768750001));
#13663=CARTESIAN_POINT('',(-28.7949008378137,169.000512499998,-140.625768750001));
#13664=CARTESIAN_POINT('',(-80.5957703324788,98.5672184524782,-46.904030908994));
#13665=CARTESIAN_POINT('',(-80.5957703324788,98.567218452478,-46.9040309089941));
#13666=CARTESIAN_POINT('',(-82.595770332479,105.495421682753,-43.4399292938557));
#13667=CARTESIAN_POINT('Ctrl Pts',(-80.5957703324787,98.5672184524781,-46.9040309089941));
#13668=CARTESIAN_POINT('Ctrl Pts',(-80.1583076046396,98.5672184524781,-46.6514616853158));
#13669=CARTESIAN_POINT('Ctrl Pts',(-79.731847375509,98.6399471087077,-46.316319579711));
#13670=CARTESIAN_POINT('Ctrl Pts',(-79.0280064685973,98.9402745490956,-45.5660699284182));
#13671=CARTESIAN_POINT('Ctrl Pts',(-78.7496249554672,99.168633673537,-45.1522067177974));
#13672=CARTESIAN_POINT('Ctrl Pts',(-78.3748022679429,99.7108672272503,-44.3867423304201));
#13673=CARTESIAN_POINT('Ctrl Pts',(-78.2527827584179,100.061688880156,-43.983215927173));
#13674=CARTESIAN_POINT('Ctrl Pts',(-78.1901153330479,100.862134488935,-43.2736771449321));
#13675=CARTESIAN_POINT('Ctrl Pts',(-78.2490409596484,101.312629171298,-42.9686854143502));
#13676=CARTESIAN_POINT('Ctrl Pts',(-78.5015571253347,102.1873708287,-42.531314585649));
#13677=CARTESIAN_POINT('Ctrl Pts',(-78.7110997683144,102.666877512603,-42.3713056330979));
#13678=CARTESIAN_POINT('Ctrl Pts',(-79.2661565338858,103.572118612493,-42.2280010610046));
#13679=CARTESIAN_POINT('Ctrl Pts',(-79.6121998656049,103.997338243878,-42.2435068221059));
#13680=CARTESIAN_POINT('Ctrl Pts',(-80.340691634629,104.680250326612,-42.3963983912593));
#13681=CARTESIAN_POINT('Ctrl Pts',(-80.7727618736163,104.984284565641,-42.5440649201448));
#13682=CARTESIAN_POINT('Ctrl Pts',(-81.6811020778789,105.3923634715,-42.9401113983139));
#13683=CARTESIAN_POINT('Ctrl Pts',(-82.15830760464,105.495421682753,-43.1873600701774));
#13684=CARTESIAN_POINT('Ctrl Pts',(-82.595770332479,105.495421682753,-43.4399292938557));
#13685=CARTESIAN_POINT('',(-82.595770332479,105.495421682753,-43.4399292938557));
#13686=CARTESIAN_POINT('Origin',(-66.9004624423481,99.0000000000011,-70.6249999999998));
#13687=CARTESIAN_POINT('',(-69.4985386537014,96.000000000001,-70.1249999999998));
#13688=CARTESIAN_POINT('Origin',(-66.9004624423481,99.0000000000011,-70.6249999999998));
#13689=CARTESIAN_POINT('',(-69.1737791272823,96.375000000001,-70.1874999999998));
#13690=CARTESIAN_POINT('Origin',(-66.9004624423481,99.0000000000011,-70.6249999999998));
#13691=CARTESIAN_POINT('Origin',(-124.924608333924,166.000512500002,29.8757687500004));
#13692=CARTESIAN_POINT('',(-127.522684545277,163.000512500001,30.3757687500005));
#13693=CARTESIAN_POINT('',(-68.5256626279059,105.495421682756,-67.8100707061432));
#13694=CARTESIAN_POINT('',(-68.5256626279059,105.495421682756,-67.8100707061433));
#13695=CARTESIAN_POINT('',(-70.5256626279056,98.5672184524799,-64.3459690910059));
#13696=CARTESIAN_POINT('Ctrl Pts',(-68.5256626279059,105.495421682756,-67.8100707061432));
#13697=CARTESIAN_POINT('Ctrl Pts',(-68.0881999000668,105.495421682756,-67.5575014824649));
#13698=CARTESIAN_POINT('Ctrl Pts',(-67.6354735058005,105.392363471503,-67.2678537093952));
#13699=CARTESIAN_POINT('Ctrl Pts',(-66.8383170924954,104.984284565643,-66.6792312563097));
#13700=CARTESIAN_POINT('Ctrl Pts',(-66.4943990076982,104.680250326615,-66.3788807175702));
#13701=CARTESIAN_POINT('Ctrl Pts',(-65.9977451402748,103.99733824388,-65.8244341237244));
#13702=CARTESIAN_POINT('Ctrl Pts',(-65.8112950913965,103.572118612495,-65.5325046881962));
#13703=CARTESIAN_POINT('Ctrl Pts',(-65.657872108522,102.666877512605,-64.9801591426223));
#13704=CARTESIAN_POINT('Ctrl Pts',(-65.6916726047743,102.187370828702,-64.7186854143503));
#13705=CARTESIAN_POINT('Ctrl Pts',(-65.9441887704605,101.3126291713,-64.2813145856493));
#13706=CARTESIAN_POINT('Ctrl Pts',(-66.1788565437883,100.862134488937,-64.0777876307885));
#13707=CARTESIAN_POINT('Ctrl Pts',(-66.8246688668641,100.061688880158,-63.7772898220283));
#13708=CARTESIAN_POINT('Ctrl Pts',(-67.2351427379364,99.7108672272523,-63.6811986154108));
#13709=CARTESIAN_POINT('Ctrl Pts',(-68.0854656868595,99.1686336735389,-63.623072391033));
#13710=CARTESIAN_POINT('Ctrl Pts',(-68.5830724975138,98.9402745490975,-63.6572262480373));
#13711=CARTESIAN_POINT('Ctrl Pts',(-69.5847282081697,98.6399471087095,-63.8916455279991));
#13712=CARTESIAN_POINT('Ctrl Pts',(-70.0881999000665,98.5672184524799,-64.0933998673275));
#13713=CARTESIAN_POINT('Ctrl Pts',(-70.5256626279056,98.5672184524799,-64.3459690910059));
#13714=CARTESIAN_POINT('',(-70.5256626279056,98.5672184524799,-64.3459690910059));
#13715=CARTESIAN_POINT('Origin',(-96.4746890553668,99.4494897427822,-48.5986671816671));
#13716=CARTESIAN_POINT('',(-94.430917460329,100.684620539947,-45.3897032396429));
#13717=CARTESIAN_POINT('Origin',(-96.4746890553668,99.4494897427822,-48.5986671816671));
#13718=CARTESIAN_POINT('',(-94.6863889097089,100.530229190302,-45.7908237323958));
#13719=CARTESIAN_POINT('Origin',(-96.4746890553669,99.4494897427822,-48.598667181667));
#13720=CARTESIAN_POINT('Origin',(41.8109368646032,203.413715679656,-176.687875705469));
#13721=CARTESIAN_POINT('',(43.8547084596409,204.648846476821,-173.478911763445));
#13722=CARTESIAN_POINT('Origin',(-79.9327200516597,99.449489742784,-77.250197953318));
#13723=CARTESIAN_POINT('',(-77.1059069082159,97.3101804481012,-75.3975017575705));
#13724=CARTESIAN_POINT('Origin',(-79.9327200516597,99.449489742784,-77.250197953318));
#13725=CARTESIAN_POINT('',(-77.4592585511463,97.5775941099365,-75.629088782039));
#13726=CARTESIAN_POINT('Origin',(-79.9327200516597,99.4494897427839,-77.250197953318));
#13727=CARTESIAN_POINT('Origin',(-121.718415623925,203.413715679661,106.553271333508));
#13728=CARTESIAN_POINT('',(-118.891602480482,201.274406384978,108.405967529256));
#13729=CARTESIAN_POINT('Origin',(-108.737631016432,99.7320508075681,-56.2438021535162));
#13730=CARTESIAN_POINT('',(-107.276159708174,100.386816955051,-52.5783713592919));
#13731=CARTESIAN_POINT('Origin',(-108.737631016432,99.7320508075681,-56.2438021535162));
#13732=CARTESIAN_POINT('',(-107.458843621706,100.304971186616,-53.03655020857));
#13733=CARTESIAN_POINT('Origin',(-108.737631016432,99.732050807568,-56.2438021535162));
#13734=CARTESIAN_POINT('Origin',(125.171333134686,225.083486900949,-171.899270921774));
#13735=CARTESIAN_POINT('',(126.632804442944,225.738253048432,-168.23384012755));
#13736=CARTESIAN_POINT('Origin',(-92.6850721331748,99.7320508075696,-84.0476497308099));
#13737=CARTESIAN_POINT('',(-89.6744074864335,97.2884302780867,-83.0655005095853));
#13738=CARTESIAN_POINT('Origin',(-92.6850721331748,99.7320508075696,-84.0476497308099));
#13739=CARTESIAN_POINT('',(-90.0507405672762,97.5938828442721,-83.1882691622385));
#13740=CARTESIAN_POINT('Origin',(-92.6850721331748,99.7320508075696,-84.0476497308099));
#13741=CARTESIAN_POINT('Origin',(-75.8911640975186,225.083486900956,176.351189781088));
#13742=CARTESIAN_POINT('',(-72.8804994507773,222.639866371473,177.333339002313));
#13743=CARTESIAN_POINT('Origin',(-121.472809584586,99.8284271247455,-63.7892135623721));
#13744=CARTESIAN_POINT('',(-120.716880638568,99.8284271247455,-59.8612915381242));
#13745=CARTESIAN_POINT('Origin',(-121.472809584586,99.8284271247455,-63.7892135623721));
#13746=CARTESIAN_POINT('',(-120.81137175682,99.8284271247455,-60.3522817911552));
#13747=CARTESIAN_POINT('Origin',(-121.472809584586,99.8284271247455,-63.7892135623721));
#13748=CARTESIAN_POINT('Origin',(201.051502502506,223.968092727195,-125.859046363603));
#13749=CARTESIAN_POINT('',(201.807431448525,223.968092727195,-121.931124339356));
#13750=CARTESIAN_POINT('Origin',(-105.587179379326,99.8284271247468,-91.303932188134));
#13751=CARTESIAN_POINT('',(-102.563463595252,97.2098124419149,-91.303932188134));
#13752=CARTESIAN_POINT('Origin',(-105.587179379326,99.8284271247468,-91.303932188134));
#13753=CARTESIAN_POINT('',(-102.941428068262,97.5371392772689,-91.303932188134));
#13754=CARTESIAN_POINT('Origin',(-105.587179379326,99.8284271247468,-91.303932188134));
#13755=CARTESIAN_POINT('Origin',(1.92092464970915,223.968092727204,219.045231817999));
#13756=CARTESIAN_POINT('',(4.94464043378298,221.349478044372,219.045231817999));
#13757=CARTESIAN_POINT('Origin',(-74.2616783745156,107.500000000001,-57.8749999999998));
#13758=CARTESIAN_POINT('',(-70.018153895972,98.4000000000012,-68.0249999999999));
#13759=CARTESIAN_POINT('',(-76.080331722463,105.400000000001,-57.5249999999998));
#13760=CARTESIAN_POINT('Origin',(-68.1995005480246,100.500000000001,-68.3749999999999));
#13761=CARTESIAN_POINT('Origin',(-76.8597545858689,107.499999999999,-53.3749999999998));
#13762=CARTESIAN_POINT('',(-84.7405857603073,102.599999999999,-42.5249999999996));
#13763=CARTESIAN_POINT('',(-78.6784079338163,109.599999999999,-53.0249999999997));
#13764=CARTESIAN_POINT('Origin',(-82.9219324123599,100.499999999999,-42.8749999999997));
#13765=CARTESIAN_POINT('Origin',(-83.2326628767165,107.659859266241,-62.734681784761));
#13766=CARTESIAN_POINT('',(-78.5362937027295,99.4008619759398,-73.3917489394908));
#13767=CARTESIAN_POINT('',(-81.2538936763059,106.162342759963,-61.4377944477378));
#13768=CARTESIAN_POINT('Origin',(-80.5150629031402,100.898378482218,-74.6886362765139));
#13769=CARTESIAN_POINT('Origin',(-85.5538547168813,107.659859266239,-58.7142595834813));
#13770=CARTESIAN_POINT('',(-93.1168428791077,101.762970040231,-48.1374969637468));
#13771=CARTESIAN_POINT('',(-84.1232146003549,108.524450824255,-56.4679848240644));
#13772=CARTESIAN_POINT('Origin',(-94.5474829956341,100.898378482216,-50.3837717231637));
#13773=CARTESIAN_POINT('Origin',(-91.6988562010068,107.093266739737,-68.7558258325585));
#13774=CARTESIAN_POINT('',(-90.4035687747792,99.3205545426085,-80.661588117438));
#13775=CARTESIAN_POINT('',(-89.5913909482879,105.3827323691,-68.0683213777014));
#13776=CARTESIAN_POINT('Origin',(-92.511034027498,101.031088913246,-81.3490925722951));
#13777=CARTESIAN_POINT('Origin',(-95.0014150842646,107.093266739736,-63.0356260517679));
#13778=CARTESIAN_POINT('',(-105.290562994975,101.489425216483,-54.8765577560743));
#13779=CARTESIAN_POINT('',(-93.9783851684838,107.551603042974,-60.469824495811));
#13780=CARTESIAN_POINT('Origin',(-106.313592910756,101.031088913245,-57.4423593120313));
#13781=CARTESIAN_POINT('Origin',(-100.382013675912,105.838834764833,-76.2779130879201));
#13782=CARTESIAN_POINT('',(-102.552019676931,99.0560570185445,-88.6522817586846));
#13783=CARTESIAN_POINT('',(-98.2654126270599,104.00580448685,-76.2779130879202));
#13784=CARTESIAN_POINT('Origin',(-104.668620725782,100.889087296527,-88.6522817586846));
#13785=CARTESIAN_POINT('Origin',(-105.857312474343,105.838834764831,-66.7944173824152));
#13786=CARTESIAN_POINT('',(-118.187983361742,100.889087296525,-61.5699982312887));
#13787=CARTESIAN_POINT('',(-105.328162212131,105.838834764831,-64.0448719654417));
#13788=CARTESIAN_POINT('Origin',(-118.717133623955,100.889087296525,-64.3195436482622));
#13789=CARTESIAN_POINT('Origin',(-82.9219324123599,100.499999999999,-42.8749999999996));
#13790=CARTESIAN_POINT('',(-85.1952490972941,103.124999999999,-42.4374999999996));
#13791=CARTESIAN_POINT('Origin',(-82.9219324123599,100.499999999999,-42.8749999999996));
#13792=CARTESIAN_POINT('Origin',(-82.9219324123599,100.499999999999,-42.8749999999996));
#13793=CARTESIAN_POINT('',(-85.1952490972941,103.124999999999,-42.4374999999996));
#13794=CARTESIAN_POINT('Origin',(-68.1995005480247,100.500000000001,-68.3749999999998));
#13795=CARTESIAN_POINT('',(-70.4728172329589,97.875000000001,-67.9374999999998));
#13796=CARTESIAN_POINT('Origin',(-68.1995005480247,100.500000000001,-68.3749999999998));
#13797=CARTESIAN_POINT('Origin',(-68.1995005480247,100.500000000001,-68.3749999999998));
#13798=CARTESIAN_POINT('',(-70.4728172329589,97.875000000001,-67.9374999999998));
#13799=CARTESIAN_POINT('Origin',(-94.5474829956341,100.898378482216,-50.3837717231636));
#13800=CARTESIAN_POINT('',(-92.7591828499761,101.979117929735,-47.5759282738925));
#13801=CARTESIAN_POINT('Origin',(-94.5474829956341,100.898378482216,-50.3837717231636));
#13802=CARTESIAN_POINT('Origin',(-94.5474829956341,100.898378482216,-50.3837717231636));
#13803=CARTESIAN_POINT('',(-92.7591828499761,101.979117929735,-47.5759282738925));
#13804=CARTESIAN_POINT('Origin',(-80.5150629031403,100.898378482218,-74.6886362765138));
#13805=CARTESIAN_POINT('',(-78.041601402627,99.0264828493701,-73.0675271052348));
#13806=CARTESIAN_POINT('Origin',(-80.5150629031403,100.898378482218,-74.6886362765138));
#13807=CARTESIAN_POINT('Origin',(-80.5150629031403,100.898378482218,-74.6886362765138));
#13808=CARTESIAN_POINT('',(-78.041601402627,99.0264828493701,-73.0675271052348));
#13809=CARTESIAN_POINT('Origin',(-106.313592910756,101.031088913245,-57.4423593120312));
#13810=CARTESIAN_POINT('',(-105.03480551603,101.604009292292,-54.235107367085));
#13811=CARTESIAN_POINT('Origin',(-106.313592910756,101.031088913245,-57.4423593120312));
#13812=CARTESIAN_POINT('Origin',(-106.313592910756,101.031088913245,-57.4423593120312));
#13813=CARTESIAN_POINT('',(-105.03480551603,101.604009292292,-54.235107367085));
#13814=CARTESIAN_POINT('Origin',(-92.5110340274981,101.031088913246,-81.349092572295));
#13815=CARTESIAN_POINT('',(-89.8767024615995,98.8929209499488,-80.4897120037236));
#13816=CARTESIAN_POINT('Origin',(-92.5110340274981,101.031088913246,-81.349092572295));
#13817=CARTESIAN_POINT('Origin',(-92.5110340274981,101.031088913246,-81.349092572295));
#13818=CARTESIAN_POINT('',(-89.8767024615995,98.8929209499488,-80.4897120037236));
#13819=CARTESIAN_POINT('Origin',(-118.717133623955,100.889087296525,-64.319543648262));
#13820=CARTESIAN_POINT('',(-118.055695796189,100.889087296525,-60.8826118770452));
#13821=CARTESIAN_POINT('Origin',(-118.717133623955,100.889087296525,-64.319543648262));
#13822=CARTESIAN_POINT('Origin',(-118.717133623955,100.889087296525,-64.319543648262));
#13823=CARTESIAN_POINT('',(-118.055695796189,100.889087296525,-60.8826118770452));
#13824=CARTESIAN_POINT('Origin',(-104.668620725782,100.889087296527,-88.6522817586845));
#13825=CARTESIAN_POINT('',(-102.022869414718,98.5977994490487,-88.6522817586845));
#13826=CARTESIAN_POINT('Origin',(-104.668620725782,100.889087296527,-88.6522817586845));
#13827=CARTESIAN_POINT('Origin',(-104.668620725782,100.889087296527,-88.6522817586845));
#13828=CARTESIAN_POINT('',(-102.022869414718,98.5977994490487,-88.6522817586845));
#13829=CARTESIAN_POINT('Origin',(-125.268934230709,90.999,-76.5975199760558));
#13830=CARTESIAN_POINT('',(-122.424179917669,121.863728726179,-74.9551003076436));
#13831=CARTESIAN_POINT('Origin',(-118.577560436093,90.999,-88.1873193607661));
#13832=CARTESIAN_POINT('',(-115.732806123053,121.863728726179,-86.5448996923539));
#13833=CARTESIAN_POINT('Origin',(-115.529994481957,90.999,-74.0824712601139));
#13834=CARTESIAN_POINT('',(-115.529994481957,122.937359864766,-74.0824712601139));
#13835=CARTESIAN_POINT('',(-115.529994481957,122.937359864766,-74.0824712601139));
#13836=CARTESIAN_POINT('',(-115.529994481957,122.937359864766,-74.082471260114));
#13837=CARTESIAN_POINT('Origin',(-111.529994481957,90.999,-81.0106744903897));
#13838=CARTESIAN_POINT('',(-111.529994481957,122.937359864767,-81.0106744903897));
#13839=CARTESIAN_POINT('',(-111.529994481957,122.937359864767,-81.0106744903897));
#13840=CARTESIAN_POINT('',(-111.529994481957,122.937359864767,-81.0106744903897));
#13841=CARTESIAN_POINT('Ctrl Pts',(-111.529994481957,122.930969193824,-81.0106744903897));
#13842=CARTESIAN_POINT('Ctrl Pts',(-111.529994481957,124.224440992555,-81.0106744903897));
#13843=CARTESIAN_POINT('Ctrl Pts',(-111.850631939497,122.930969193824,-81.1957946128129));
#13844=CARTESIAN_POINT('Ctrl Pts',(-111.850631939497,124.224440992555,-81.1957946128129));
#13845=CARTESIAN_POINT('Ctrl Pts',(-112.595893637265,122.930969193824,-81.3855792709696));
#13846=CARTESIAN_POINT('Ctrl Pts',(-112.595893637265,124.224440992555,-81.3855792709696));
#13847=CARTESIAN_POINT('Ctrl Pts',(-113.856111715799,122.930969193824,-81.0858699693662));
#13848=CARTESIAN_POINT('Ctrl Pts',(-113.856111715799,124.224440992555,-81.0858699693662));
#13849=CARTESIAN_POINT('Ctrl Pts',(-115.066649862454,122.930969193824,-80.2473165597762));
#13850=CARTESIAN_POINT('Ctrl Pts',(-115.066649862454,124.224440992555,-80.2473165597762));
#13851=CARTESIAN_POINT('Ctrl Pts',(-116.043255168468,122.930969193824,-78.9976046091529));
#13852=CARTESIAN_POINT('Ctrl Pts',(-116.043255168468,124.224440992555,-78.9976046091529));
#13853=CARTESIAN_POINT('Ctrl Pts',(-116.637234812114,122.930969193824,-77.5269836293621));
#13854=CARTESIAN_POINT('Ctrl Pts',(-116.637234812114,124.224440992555,-77.5269836293621));
#13855=CARTESIAN_POINT('Ctrl Pts',(-116.758174293921,122.930969193824,-76.0593501373141));
#13856=CARTESIAN_POINT('Ctrl Pts',(-116.758174293921,124.224440992555,-76.0593501373141));
#13857=CARTESIAN_POINT('Ctrl Pts',(-116.387621123593,122.930969193824,-74.8181146161938));
#13858=CARTESIAN_POINT('Ctrl Pts',(-116.387621123593,124.224440992555,-74.8181146161938));
#13859=CARTESIAN_POINT('Ctrl Pts',(-115.850631939497,122.930969193824,-74.2675913825374));
#13860=CARTESIAN_POINT('Ctrl Pts',(-115.850631939497,124.224440992555,-74.2675913825374));
#13861=CARTESIAN_POINT('Ctrl Pts',(-115.529994481957,122.930969193824,-74.0824712601142));
#13862=CARTESIAN_POINT('Ctrl Pts',(-115.529994481957,124.224440992555,-74.0824712601142));
#13863=CARTESIAN_POINT('Ctrl Pts',(-111.529994481957,122.937359864767,-81.0106744903897));
#13864=CARTESIAN_POINT('Ctrl Pts',(-111.655985564703,122.937359864767,-81.0834154759286));
#13865=CARTESIAN_POINT('Ctrl Pts',(-111.789124566157,122.941999166342,-81.1417276437762));
#13866=CARTESIAN_POINT('Ctrl Pts',(-112.132055648316,122.963800802529,-81.2508717728567));
#13867=CARTESIAN_POINT('Ctrl Pts',(-112.344262065112,122.985642902608,-81.2836304965519));
#13868=CARTESIAN_POINT('Ctrl Pts',(-112.890185001658,123.055781639719,-81.2942385303482));
#13869=CARTESIAN_POINT('Ctrl Pts',(-113.222304091371,123.111288356191,-81.2310605511146));
#13870=CARTESIAN_POINT('Ctrl Pts',(-114.040071204807,123.254369388729,-80.9469153854904));
#13871=CARTESIAN_POINT('Ctrl Pts',(-114.507617463249,123.341916036999,-80.64733737895));
#13872=CARTESIAN_POINT('Ctrl Pts',(-115.174813131733,123.441390970383,-80.050767705693));
#13873=CARTESIAN_POINT('Ctrl Pts',(-115.415868442681,123.470261290121,-79.7826739036937));
#13874=CARTESIAN_POINT('Ctrl Pts',(-115.755003463233,123.495239476746,-79.3250674771333));
#13875=CARTESIAN_POINT('Ctrl Pts',(-115.872462661464,123.49998997396,-79.1461011463315));
#13876=CARTESIAN_POINT('Ctrl Pts',(-116.085775238015,123.500009989414,-78.7767368883965));
#13877=CARTESIAN_POINT('Ctrl Pts',(-116.182038306449,123.495284034831,-78.5856508621904));
#13878=CARTESIAN_POINT('Ctrl Pts',(-116.408570505306,123.47040914673,-78.0640352851986));
#13879=CARTESIAN_POINT('Ctrl Pts',(-116.52014584973,123.4416707474,-77.7220494143149));
#13880=CARTESIAN_POINT('Ctrl Pts',(-116.700435952419,123.344280060835,-76.8627043141552));
#13881=CARTESIAN_POINT('Ctrl Pts',(-116.72827833538,123.260349185246,-76.3253510567926));
#13882=CARTESIAN_POINT('Ctrl Pts',(-116.580959608512,123.119417363555,-75.4852207472909));
#13883=CARTESIAN_POINT('Ctrl Pts',(-116.473976785389,123.063000944788,-75.16186977102));
#13884=CARTESIAN_POINT('Ctrl Pts',(-116.194331351315,122.989309527258,-74.6783741194887));
#13885=CARTESIAN_POINT('Ctrl Pts',(-116.055391044604,122.965592809847,-74.5005585112936));
#13886=CARTESIAN_POINT('Ctrl Pts',(-115.831958999688,122.946686478982,-74.2944546113625));
#13887=CARTESIAN_POINT('Ctrl Pts',(-115.771332129154,122.942999951482,-74.2445494425702));
#13888=CARTESIAN_POINT('Ctrl Pts',(-115.650653287831,122.938455031077,-74.1565333304243));
#13889=CARTESIAN_POINT('Ctrl Pts',(-115.591330433288,122.937359864766,-74.1178835881261));
#13890=CARTESIAN_POINT('Ctrl Pts',(-115.529994481957,122.937359864766,-74.0824712601142));
#13891=CARTESIAN_POINT('Origin',(-119.078493020361,109.,-80.7499999999988));
#13892=CARTESIAN_POINT('Origin',(-141.995606772677,139.904097174214,-47.6260732918001));
#13893=CARTESIAN_POINT('',(-111.835491639576,108.363035329266,-93.2952463908106));
#13894=CARTESIAN_POINT('Origin',(-145.341293669985,128.314297789504,-41.8311735994448));
#13895=CARTESIAN_POINT('',(-115.181178536884,96.7732359445553,-87.5003466984555));
#13896=CARTESIAN_POINT('Origin',(-134.275197369886,137.573299096998,-41.6148274600336));
#13897=CARTESIAN_POINT('',(-106.49494062967,105.495421682756,-89.7316435813967));
#13898=CARTESIAN_POINT('',(-106.49494062967,105.495421682756,-89.7316435813967));
#13899=CARTESIAN_POINT('',(-106.49494062967,105.495421682756,-89.7316435813966));
#13900=CARTESIAN_POINT('Origin',(-136.275197369886,130.645095866722,-38.1507258448956));
#13901=CARTESIAN_POINT('',(-108.494940629669,98.5672184524796,-86.2675419662591));
#13902=CARTESIAN_POINT('',(-108.494940629669,98.5672184524796,-86.2675419662591));
#13903=CARTESIAN_POINT('',(-108.494940629669,98.5672184524797,-86.2675419662591));
#13904=CARTESIAN_POINT('Ctrl Pts',(-108.497707871361,98.5704137879512,-86.2627489630519));
#13905=CARTESIAN_POINT('Ctrl Pts',(-107.937618152971,97.9236778885854,-87.2328528121005));
#13906=CARTESIAN_POINT('Ctrl Pts',(-108.818345328902,98.5704137879512,-86.4478690854752));
#13907=CARTESIAN_POINT('Ctrl Pts',(-108.258255610512,97.9236778885854,-87.4179729345238));
#13908=CARTESIAN_POINT('Ctrl Pts',(-109.407402641416,98.750783075701,-86.9082076752565));
#13909=CARTESIAN_POINT('Ctrl Pts',(-108.847312923026,98.1040471763352,-87.8783115243051));
#13910=CARTESIAN_POINT('Ctrl Pts',(-110.000372038795,99.5212554870629,-87.7642069906961));
#13911=CARTESIAN_POINT('Ctrl Pts',(-109.440282320405,98.8745195876971,-88.7343108397447));
#13912=CARTESIAN_POINT('Ctrl Pts',(-110.212301964103,100.674348937882,-88.6552937573345));
#13913=CARTESIAN_POINT('Ctrl Pts',(-109.652212245713,100.027613038516,-89.6253976063831));
#13914=CARTESIAN_POINT('Ctrl Pts',(-110.010968557873,102.034515403089,-89.4458315045219));
#13915=CARTESIAN_POINT('Ctrl Pts',(-109.450878839483,101.387779503723,-90.4159353535705));
#13916=CARTESIAN_POINT('Ctrl Pts',(-109.427009489273,103.394681868296,-90.0154602225416));
#13917=CARTESIAN_POINT('Ctrl Pts',(-108.866919770883,102.74794596893,-90.9855640715902));
#13918=CARTESIAN_POINT('Ctrl Pts',(-108.549340749734,104.547775319115,-90.2774669067221));
#13919=CARTESIAN_POINT('Ctrl Pts',(-107.989251031344,103.901039419749,-91.2475707557707));
#13920=CARTESIAN_POINT('Ctrl Pts',(-107.511538898252,105.318247730477,-90.1919400026446));
#13921=CARTESIAN_POINT('Ctrl Pts',(-106.951449179862,104.671511831111,-91.1620438516932));
#13922=CARTESIAN_POINT('Ctrl Pts',(-106.818345328902,105.498617018227,-89.9119707006131));
#13923=CARTESIAN_POINT('Ctrl Pts',(-106.258255610512,104.851881118861,-90.8820745496617));
#13924=CARTESIAN_POINT('Ctrl Pts',(-106.497707871361,105.498617018227,-89.7268505781898));
#13925=CARTESIAN_POINT('Ctrl Pts',(-105.937618152971,104.851881118861,-90.6969544272384));
#13926=CARTESIAN_POINT('Ctrl Pts',(-108.494940629669,98.5672184524797,-86.2675419662592));
#13927=CARTESIAN_POINT('Ctrl Pts',(-108.620931712415,98.5672184524797,-86.3402829517981));
#13928=CARTESIAN_POINT('Ctrl Pts',(-108.740009575843,98.5788155545531,-86.4229497251191));
#13929=CARTESIAN_POINT('Ctrl Pts',(-109.015792308145,98.634550154098,-86.6483982077968));
#13930=CARTESIAN_POINT('Ctrl Pts',(-109.160240827059,98.6909481351825,-86.7985170532378));
#13931=CARTESIAN_POINT('Ctrl Pts',(-109.477961818401,98.884314307059,-87.2043824505149));
#13932=CARTESIAN_POINT('Ctrl Pts',(-109.620465834967,99.047756217635,-87.4696274118531));
#13933=CARTESIAN_POINT('Ctrl Pts',(-109.88505667753,99.5434281228911,-88.1436116529208));
#13934=CARTESIAN_POINT('Ctrl Pts',(-109.944782655288,99.9267917722889,-88.5503990928816));
#13935=CARTESIAN_POINT('Ctrl Pts',(-109.931222669289,100.613385759641,-89.132932800729));
#13936=CARTESIAN_POINT('Ctrl Pts',(-109.895248991132,100.904400962771,-89.3446672830305));
#13937=CARTESIAN_POINT('Ctrl Pts',(-109.799168414145,101.381966460934,-89.6408763836526));
#13938=CARTESIAN_POINT('Ctrl Pts',(-109.754281345734,101.564677285217,-89.7431020350957));
#13939=CARTESIAN_POINT('Ctrl Pts',(-109.647683916166,101.93405752606,-89.9278381616077));
#13940=CARTESIAN_POINT('Ctrl Pts',(-109.585780717548,102.121418154361,-90.0107041459795));
#13941=CARTESIAN_POINT('Ctrl Pts',(-109.399335228826,102.623158600648,-90.2043869062662));
#13942=CARTESIAN_POINT('Ctrl Pts',(-109.259387572093,102.942330744829,-90.2980516526588));
#13943=CARTESIAN_POINT('Ctrl Pts',(-108.856079275086,103.713602817721,-90.4495286319902));
#13944=CARTESIAN_POINT('Ctrl Pts',(-108.560802720886,104.170639304011,-90.4718337906789));
#13945=CARTESIAN_POINT('Ctrl Pts',(-107.984073142598,104.807412067022,-90.3754648931577));
#13946=CARTESIAN_POINT('Ctrl Pts',(-107.731615284225,105.031808587313,-90.3040840691712));
#13947=CARTESIAN_POINT('Ctrl Pts',(-107.274706570105,105.310186009746,-90.1276174249943));
#13948=CARTESIAN_POINT('Ctrl Pts',(-107.082643892882,105.395243156987,-90.0418124615454));
#13949=CARTESIAN_POINT('Ctrl Pts',(-106.81731713635,105.462525333909,-89.9082723306999));
#13950=CARTESIAN_POINT('Ctrl Pts',(-106.748607297535,105.475545269237,-89.8723672736483));
#13951=CARTESIAN_POINT('Ctrl Pts',(-106.617982888177,105.491574342406,-89.8015773906488));
#13952=CARTESIAN_POINT('Ctrl Pts',(-106.556276581001,105.495421682755,-89.7670559094086));
#13953=CARTESIAN_POINT('Ctrl Pts',(-106.49494062967,105.495421682755,-89.7316435813966));
#13954=CARTESIAN_POINT('Origin',(-119.078493020361,109.,-80.7499999999988));
#13955=CARTESIAN_POINT('Origin',(-98.8802009968175,127.881285087611,-122.304146684539));
#13956=CARTESIAN_POINT('',(-122.975807503838,96.7732359445554,-73.9996533015419));
#13957=CARTESIAN_POINT('Origin',(-102.225887894125,139.471084472322,-116.509246992184));
#13958=CARTESIAN_POINT('',(-126.321494401146,108.363035329266,-68.2047536091869));
#13959=CARTESIAN_POINT('Origin',(-91.1597915940262,130.212083164828,-116.292900852773));
#13960=CARTESIAN_POINT('',(-118.565048334243,98.5672184524784,-68.8256037842474));
#13961=CARTESIAN_POINT('',(-118.565048334243,98.5672184524783,-68.8256037842474));
#13962=CARTESIAN_POINT('',(-118.565048334243,98.5672184524784,-68.8256037842474));
#13963=CARTESIAN_POINT('Origin',(-93.159791594026,137.140286395103,-112.828799237635));
#13964=CARTESIAN_POINT('',(-120.565048334243,105.495421682754,-65.3615021691091));
#13965=CARTESIAN_POINT('',(-120.565048334243,105.495421682754,-65.3615021691091));
#13966=CARTESIAN_POINT('',(-120.565048334243,105.495421682754,-65.3615021691091));
#13967=CARTESIAN_POINT('Ctrl Pts',(-120.562281092551,105.498617018225,-65.3662951723163));
#13968=CARTESIAN_POINT('Ctrl Pts',(-121.122370810941,104.85188111886,-64.3961913232677));
#13969=CARTESIAN_POINT('Ctrl Pts',(-120.882918550091,105.498617018225,-65.5514152947396));
#13970=CARTESIAN_POINT('Ctrl Pts',(-121.443008268481,104.85188111886,-64.581311445691));
#13971=CARTESIAN_POINT('Ctrl Pts',(-121.471975862605,105.318247730476,-66.0117538845209));
#13972=CARTESIAN_POINT('Ctrl Pts',(-122.032065580995,104.67151183111,-65.0416500354723));
#13973=CARTESIAN_POINT('Ctrl Pts',(-122.064945259985,104.547775319114,-66.8677531999604));
#13974=CARTESIAN_POINT('Ctrl Pts',(-122.625034978375,103.901039419748,-65.8976493509118));
#13975=CARTESIAN_POINT('Ctrl Pts',(-122.276875185293,103.394681868295,-67.7588399665989));
#13976=CARTESIAN_POINT('Ctrl Pts',(-122.836964903683,102.747945968929,-66.7887361175503));
#13977=CARTESIAN_POINT('Ctrl Pts',(-122.075541779062,102.034515403088,-68.5493777137862));
#13978=CARTESIAN_POINT('Ctrl Pts',(-122.635631497452,101.387779503722,-67.5792738647376));
#13979=CARTESIAN_POINT('Ctrl Pts',(-121.491582710463,100.674348937881,-69.1190064318059));
#13980=CARTESIAN_POINT('Ctrl Pts',(-122.051672428853,100.027613038515,-68.1489025827573));
#13981=CARTESIAN_POINT('Ctrl Pts',(-120.613913970924,99.5212554870615,-69.3810131159864));
#13982=CARTESIAN_POINT('Ctrl Pts',(-121.174003689314,98.8745195876958,-68.4109092669378));
#13983=CARTESIAN_POINT('Ctrl Pts',(-119.576112119442,98.7507830756997,-69.2954862119089));
#13984=CARTESIAN_POINT('Ctrl Pts',(-120.136201837832,98.104047176334,-68.3253823628603));
#13985=CARTESIAN_POINT('Ctrl Pts',(-118.882918550091,98.5704137879498,-69.0155169098773));
#13986=CARTESIAN_POINT('Ctrl Pts',(-119.443008268481,97.9236778885841,-68.0454130608287));
#13987=CARTESIAN_POINT('Ctrl Pts',(-118.562281092551,98.5704137879498,-68.8303967874541));
#13988=CARTESIAN_POINT('Ctrl Pts',(-119.122370810941,97.9236778885841,-67.8602929384055));
#13989=CARTESIAN_POINT('Ctrl Pts',(-120.565048334243,105.495421682754,-65.3615021691091));
#13990=CARTESIAN_POINT('Ctrl Pts',(-120.691039416989,105.495421682754,-65.4342431546481));
#13991=CARTESIAN_POINT('Ctrl Pts',(-120.814135033437,105.479185279105,-65.509950975606));
#13992=CARTESIAN_POINT('Ctrl Pts',(-121.108798536521,105.401649043373,-65.7026970040038));
#13993=CARTESIAN_POINT('Ctrl Pts',(-121.272162868975,105.32340896221,-65.8200526993256));
#13994=CARTESIAN_POINT('Ctrl Pts',(-121.650625788444,105.059904053223,-66.1207099909364));
#13995=CARTESIAN_POINT('Ctrl Pts',(-121.841200031555,104.840955426175,-66.3026948775666));
#13996=CARTESIAN_POINT('Ctrl Pts',(-122.229702683097,104.20220248838,-66.7620575698267));
#13997=CARTESIAN_POINT('Ctrl Pts',(-122.365246282272,103.731292190713,-67.0375250373832));
#13998=CARTESIAN_POINT('Ctrl Pts',(-122.437834115624,102.945223269976,-67.4708463451536));
#13999=CARTESIAN_POINT('Ctrl Pts',(-122.426862867774,102.625337747109,-67.6392753478494));
#14000=CARTESIAN_POINT('Ctrl Pts',(-122.352414034946,102.122794062321,-67.8980171685339));
#14001=CARTESIAN_POINT('Ctrl Pts',(-122.311641017802,101.935332740824,-67.9931170741559));
#14002=CARTESIAN_POINT('Ctrl Pts',(-122.205060922126,101.565932484526,-68.1778231774862));
#14003=CARTESIAN_POINT('Ctrl Pts',(-122.139064926783,101.383297810808,-68.2677780937319));
#14004=CARTESIAN_POINT('Ctrl Pts',(-121.931077153049,100.906432252622,-68.4987731861706));
#14005=CARTESIAN_POINT('Ctrl Pts',(-121.766241312432,100.615998507772,-68.6355455315589));
#14006=CARTESIAN_POINT('Ctrl Pts',(-121.278590206767,99.9421171214444,-68.9331085407376));
#14007=CARTESIAN_POINT('Ctrl Pts',(-120.910627382145,99.5690115107432,-69.0813100128094));
#14008=CARTESIAN_POINT('Ctrl Pts',(-120.211847266071,99.0731705694225,-69.1963388478251));
#14009=CARTESIAN_POINT('Ctrl Pts',(-119.910531355856,98.9051904678996,-69.2095826519892));
#14010=CARTESIAN_POINT('Ctrl Pts',(-119.389804002114,98.7005044629965,-69.1436531341076));
#14011=CARTESIAN_POINT('Ctrl Pts',(-119.177202045119,98.6391640331656,-69.0934232467741));
#14012=CARTESIAN_POINT('Ctrl Pts',(-118.895501925765,98.5907881871084,-68.988242612226));
#14013=CARTESIAN_POINT('Ctrl Pts',(-118.823599460482,98.5814547792815,-68.9578673464248));
#14014=CARTESIAN_POINT('Ctrl Pts',(-118.689039034596,98.5699706265173,-68.8938948440334));
#14015=CARTESIAN_POINT('Ctrl Pts',(-118.626384285574,98.5672184524785,-68.8610161122592));
#14016=CARTESIAN_POINT('Ctrl Pts',(-118.565048334243,98.5672184524785,-68.8256037842472));
#14017=CARTESIAN_POINT('Origin',(-119.078493020361,109.,-80.7499999999988));
#14018=CARTESIAN_POINT('Origin',(-69.3034604663987,124.991664350565,-51.4350212868557));
#14019=CARTESIAN_POINT('',(-67.366968793295,124.991664350565,-50.3169872981059));
#14020=CARTESIAN_POINT('Origin',(-68.8034604663987,123.191664350565,-52.3010466906402));
#14021=CARTESIAN_POINT('',(-66.866968793295,124.991664350565,-51.1830127018903));
#14022=CARTESIAN_POINT('Origin',(-69.3034604663987,124.991664350565,-51.4350212868557));
#14023=CARTESIAN_POINT('Origin',(-76.346812504256,100.571155122824,-40.3758635351318));
#14024=CARTESIAN_POINT('',(-73.9165625814855,100.571155122824,-38.9727580880221));
#14025=CARTESIAN_POINT('Origin',(-75.81738964085,102.337180526609,-41.2928508332395));
#14026=CARTESIAN_POINT('',(-74.1665625814855,101.437180526609,-38.5397453861299));
#14027=CARTESIAN_POINT('Origin',(-76.346812504256,100.571155122824,-40.3758635351318));
#14028=CARTESIAN_POINT('Origin',(-62.497624927873,101.437180526611,-64.3633600609793));
#14029=CARTESIAN_POINT('',(-60.0673750051025,101.437180526611,-62.9602546138697));
#14030=CARTESIAN_POINT('Origin',(-63.527047791279,101.471155122826,-62.580347359087));
#14031=CARTESIAN_POINT('',(-60.3173750051025,100.571155122826,-62.5272419119774));
#14032=CARTESIAN_POINT('Origin',(-62.497624927873,101.437180526611,-64.3633600609793));
#14110=UNCERTAINTY_MEASURE_WITH_UNIT(LENGTH_MEASURE(0.01),#14126,
'DISTANCE_ACCURACY_VALUE',
'Maximum model space distance between geometric entities at asserted c
onnectivities');
#14112=UNCERTAINTY_MEASURE_WITH_UNIT(LENGTH_MEASURE(0.01),#14126,
'DISTANCE_ACCURACY_VALUE',
'Maximum model space distance between geometric entities at asserted c
onnectivities');
#14123=(
GEOMETRIC_REPRESENTATION_CONTEXT(3)
GLOBAL_UNCERTAINTY_ASSIGNED_CONTEXT((#14110))
GLOBAL_UNIT_ASSIGNED_CONTEXT((#14126,#14128,#14129))
REPRESENTATION_CONTEXT('','3D')
);
#14125=(
GEOMETRIC_REPRESENTATION_CONTEXT(3)
GLOBAL_UNCERTAINTY_ASSIGNED_CONTEXT((#14112))
GLOBAL_UNIT_ASSIGNED_CONTEXT((#14126,#14128,#14129))
REPRESENTATION_CONTEXT('','3D')
);
#14126=(
LENGTH_UNIT()
NAMED_UNIT(*)
SI_UNIT(.MILLI.,.METRE.)
);
#14128=(
NAMED_UNIT(*)
PLANE_ANGLE_UNIT()
SI_UNIT($,.RADIAN.)
);
#14129=(
NAMED_UNIT(*)
SI_UNIT($,.STERADIAN.)
SOLID_ANGLE_UNIT()
);
#14140=SHAPE_DEFINITION_REPRESENTATION(#14152,#14209);
#14152=PRODUCT_DEFINITION_SHAPE('',$,#14222);
#14209=SHAPE_REPRESENTATION('',(#6669),#14123);
#14211=PRODUCT_DEFINITION_CONTEXT('part definition',#14249,'design');
#14222=PRODUCT_DEFINITION('Sprinkler','Sprinkler',#14234,#14211);
#14234=PRODUCT_DEFINITION_FORMATION('',$,#14261);
#14249=APPLICATION_CONTEXT(
'Core Data for Automotive Mechanical Design Process');
#14250=PRODUCT_CONTEXT('part definition',#14249,'mechanical');
#14261=PRODUCT('Sprinkler','Sprinkler',$,(#14250));
#14263=PRESENTATION_STYLE_ASSIGNMENT((#14265));
#14265=SURFACE_STYLE_USAGE(.BOTH.,#14267);
#14267=SURFACE_SIDE_STYLE('',(#14269));
#14269=SURFACE_STYLE_FILL_AREA(#14271);
#14271=FILL_AREA_STYLE('Steel - Satin',(#14273));
#14273=FILL_AREA_STYLE_COLOUR('Steel - Satin',#14275);
#14275=COLOUR_RGB('Steel - Satin',0.627450980392157,0.627450980392157,0.627450980392157);
ENDSEC;
END-ISO-10303-21;
